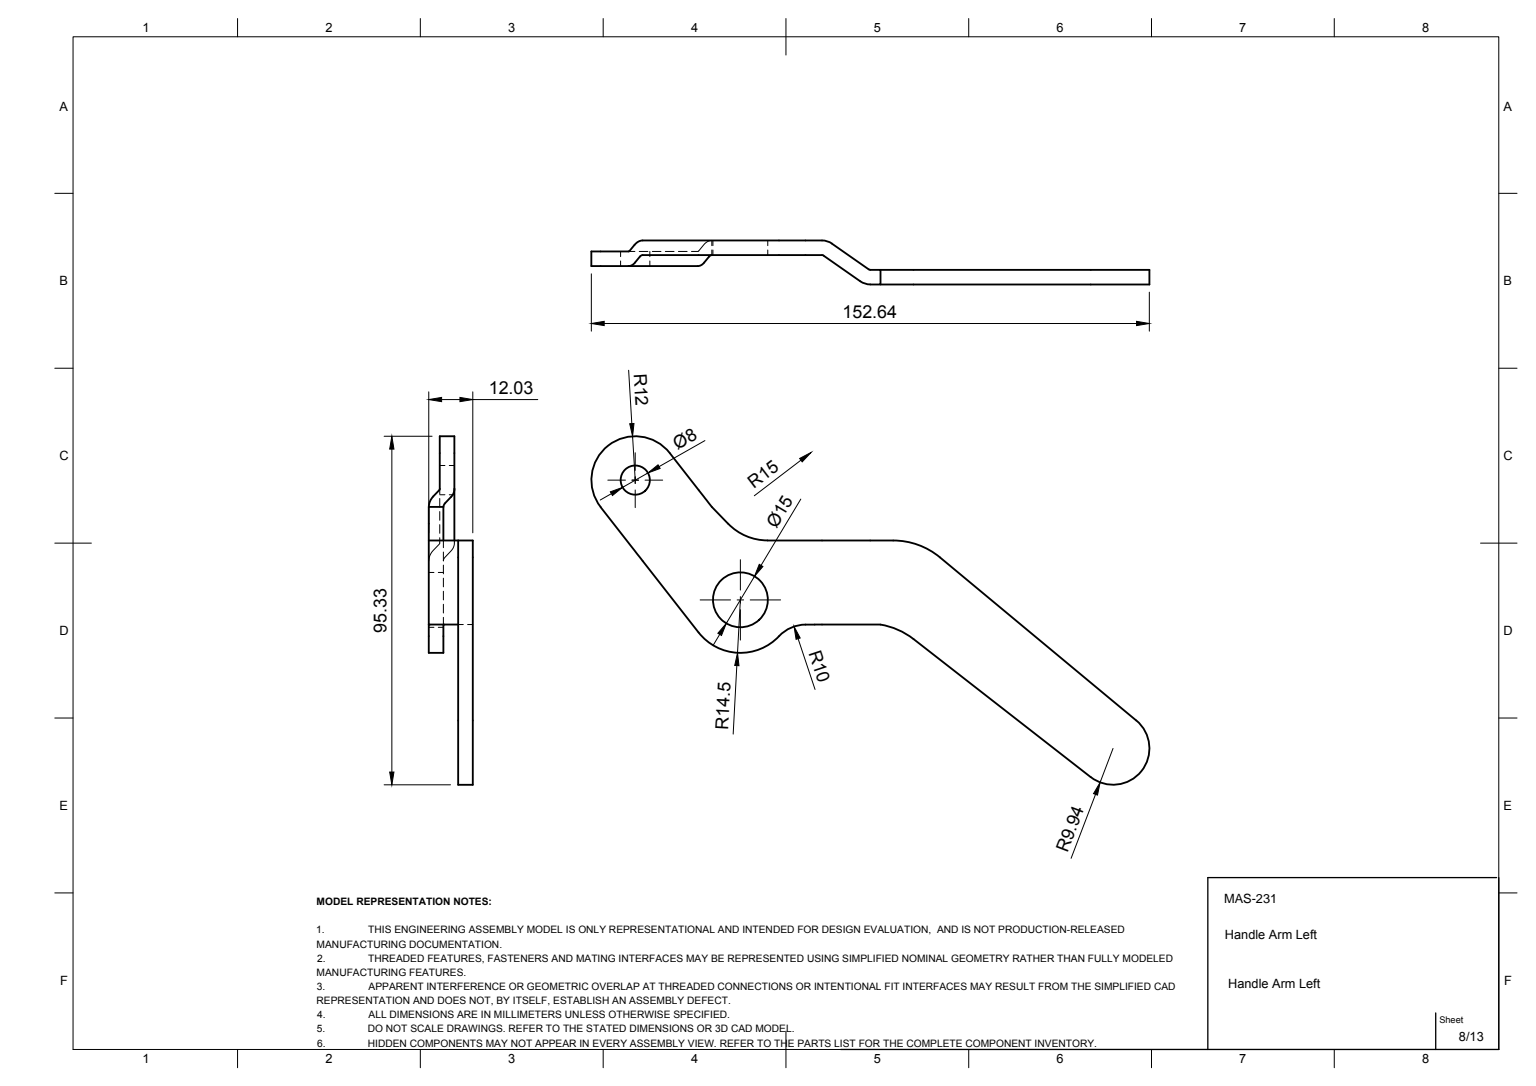
ISO-10303-21;
HEADER;
FILE_DESCRIPTION (('STEP AP214'),
    '1' );
FILE_NAME ( 'Handle Arm Left.step', '2026-10-04T02:08:54', ( '' ), ( '' ), 'STEP AP214', 'Unspecified', '' );
FILE_SCHEMA (( 'AUTOMOTIVE_DESIGN' ));
ENDSEC;
DATA;
#122=AXIS2_PLACEMENT_3D ( 'NONE', #43059, #39470, #7131 ) ;
#126=EDGE_LOOP ( 'NONE', ( #4193, #39037, #39203, #47364, #17831, #33692, #29299, #33986, #26594 ) ) ;
#187=( GEOMETRIC_REPRESENTATION_CONTEXT ( 3 ) GLOBAL_UNCERTAINTY_ASSIGNED_CONTEXT ( ( #19281 ) ) GLOBAL_UNIT_ASSIGNED_CONTEXT ( ( #14903, #26165, #18708 ) ) REPRESENTATION_CONTEXT ( 'NONE', 'WORKASPACE' ) ) ;
#223=EDGE_LOOP ( 'NONE', ( #32593, #34812, #29678, #45510 ) ) ;
#230=FACE_OUTER_BOUND ( 'NONE', #13816, .T. ) ;
#248=CARTESIAN_POINT ( 'NONE',  ( -0.3161444924769509779, 1.495705267341512767, -0.3569552279982057819 ) ) ;
#378=EDGE_CURVE ( 'NONE', #9213, #13081, #13737, .T. ) ;
#388=B_SPLINE_CURVE_WITH_KNOTS ( 'NONE', 3,
 ( #34639, #1791, #24318, #31755 ),
 .UNSPECIFIED., .F., .F.,
 ( 4, 4 ),
 ( 0.000000000000000000, 1.000000000000000000 ),
 .UNSPECIFIED. ) ;
#405=EDGE_CURVE ( 'NONE', #45750, #40086, #43961, .T. ) ;
#408=DIRECTION ( 'NONE',  ( -1.000000000000000000, 0.000000000000000000, 0.000000000000000000 ) ) ;
#422=VECTOR ( 'NONE', #8785, 39.37007874015748143 ) ;
#427=AXIS2_PLACEMENT_3D ( 'NONE', #21003, #3022, #14070 ) ;
#459=ORIENTED_EDGE ( 'NONE', *, *, #45696, .T. ) ;
#467=CARTESIAN_POINT ( 'NONE',  ( -0.07874015748031489015, -0.5708661417322835607, 0.9783464566929127582 ) ) ;
#518=CYLINDRICAL_SURFACE ( 'NONE', #9417, 0.5708661417322833387 ) ;
#533=EDGE_LOOP ( 'NONE', ( #23473, #14540, #33151, #19710 ) ) ;
#535=DIRECTION ( 'NONE',  ( 1.000000000000000000, -0.000000000000000000, -0.000000000000000000 ) ) ;
#539=CARTESIAN_POINT ( 'NONE',  ( -0.1586641775163213364, 1.209494567139720367, -1.479906699140297599 ) ) ;
#545=DIRECTION ( 'NONE',  ( 0.000000000000000000, -8.673617379884043361E-16, 1.000000000000000000 ) ) ;
#558=CARTESIAN_POINT ( 'NONE',  ( -0.1586641775163213364, 1.205832402325951680, -1.129708666049261900 ) ) ;
#616=ORIENTED_EDGE ( 'NONE', *, *, #20566, .T. ) ;
#679=FACE_OUTER_BOUND ( 'NONE', #47350, .T. ) ;
#696=AXIS2_PLACEMENT_3D ( 'NONE', #10327, #39534, #28800 ) ;
#711=AXIS2_PLACEMENT_3D ( 'NONE', #7841, #43130, #8307 ) ;
#753=EDGE_CURVE ( 'NONE', #41392, #4833, #15522, .T. ) ;
#754=PRODUCT_DEFINITION ( 'UNKNOWN', '', #15557, #11115 ) ;
#808=FACE_OUTER_BOUND ( 'NONE', #31107, .T. ) ;
#881=CARTESIAN_POINT ( 'NONE',  ( 0.1574803149606299746, 0.6241017553149654784, 0.3240160679609099259 ) ) ;
#895=CIRCLE ( 'NONE', #27749, 0.4724409448818896462 ) ;
#923=ORIENTED_EDGE ( 'NONE', *, *, #43493, .T. ) ;
#1025=ADVANCED_FACE ( 'NONE', ( #22928 ), #19568, .F. ) ;
#1029=LENGTH_MEASURE_WITH_UNIT ( LENGTH_MEASURE( 0.02539999999999999897 ), #18778 ) ;
#1037=CARTESIAN_POINT ( 'NONE',  ( -0.1184675242425147629, -0.09842519685039370636, 1.713085361781126803 ) ) ;
#1140=CARTESIAN_POINT ( 'NONE',  ( -0.3161444924769509779, 1.205832402325951680, -1.129708666049261900 ) ) ;
#1216=LINE ( 'NONE', #15633, #39726 ) ;
#1222=ORIENTED_EDGE ( 'NONE', *, *, #15124, .F. ) ;
#1296=DIRECTION ( 'NONE',  ( -0.000000000000000000, -0.2432573283306819767, 0.9699617890481142535 ) ) ;
#1309=VECTOR ( 'NONE', #45246, 39.37007874015748143 ) ;
#1316=DIRECTION ( 'NONE',  ( 0.000000000000000000, 0.000000000000000000, 1.000000000000000000 ) ) ;
#1330=LINE ( 'NONE', #2050, #12163 ) ;
#1374=DIRECTION ( 'NONE',  ( -1.000000000000000000, 0.000000000000000000, 0.000000000000000000 ) ) ;
#1393=DIRECTION ( 'NONE',  ( 0.000000000000000000, -1.000000000000000000, 0.000000000000000000 ) ) ;
#1444=EDGE_CURVE ( 'NONE', #18796, #17177, #32922, .T. ) ;
#1488=AXIS2_PLACEMENT_3D ( 'NONE', #8603, #23243, #19630 ) ;
#1493=VECTOR ( 'NONE', #28318, 39.37007874015748143 ) ;
#1494=EDGE_CURVE ( 'NONE', #3991, #16648, #40415, .T. ) ;
#1507=CARTESIAN_POINT ( 'NONE',  ( 0.03901279071809810040, -0.09842519685039370636, 1.870565676741754668 ) ) ;
#1532=EDGE_LOOP ( 'NONE', ( #26230, #3600, #16284, #44821 ) ) ;
#1601=AXIS2_PLACEMENT_3D ( 'NONE', #34251, #4042, #22736 ) ;
#1613=DIRECTION ( 'NONE',  ( 1.000000000000000000, -0.000000000000000000, -0.000000000000000000 ) ) ;
#1634=DIRECTION ( 'NONE',  ( 0.000000000000000000, 0.000000000000000000, 1.000000000000000000 ) ) ;
#1791=CARTESIAN_POINT ( 'NONE',  ( 0.1049868766404236653, 0.4668427075568369333, -0.7022306805398673690 ) ) ;
#1868=DIRECTION ( 'NONE',  ( -0.8191520442890007914, -0.4519843998600331925, 0.3531289150159138690 ) ) ;
#1878=DIRECTION ( 'NONE',  ( 0.000000000000000000, -1.000000000000000000, 0.000000000000000000 ) ) ;
#1947=EDGE_CURVE ( 'NONE', #45939, #23245, #19092, .T. ) ;
#1972=AXIS2_PLACEMENT_3D ( 'NONE', #43308, #35675, #44016 ) ;
#1994=EDGE_CURVE ( 'NONE', #30756, #31965, #2268, .T. ) ;
#2006=ORIENTED_EDGE ( 'NONE', *, *, #33798, .F. ) ;
#2044=DIRECTION ( 'NONE',  ( 0.000000000000000000, 0.000000000000000000, -1.000000000000000000 ) ) ;
#2050=CARTESIAN_POINT ( 'NONE',  ( -0.3161444924769509779, 0.8918838478058892516, -1.034309214090478823 ) ) ;
#2090=ORIENTED_EDGE ( 'NONE', *, *, #33751, .T. ) ;
#2145=DIRECTION ( 'NONE',  ( 0.000000000000000000, 0.000000000000000000, 1.000000000000000000 ) ) ;
#2163=LINE ( 'NONE', #46478, #34704 ) ;
#2207=LINE ( 'NONE', #37047, #4035 ) ;
#2248=ORIENTED_EDGE ( 'NONE', *, *, #47327, .F. ) ;
#2268=CIRCLE ( 'NONE', #24483, 0.2952755905511806334 ) ;
#2320=EDGE_CURVE ( 'NONE', #11282, #39413, #6695, .T. ) ;
#2339=CARTESIAN_POINT ( 'NONE',  ( -0.1586641775163213364, 1.975221432870719385, -0.9622519263226601005 ) ) ;
#2340=DIRECTION ( 'NONE',  ( 1.000000000000000000, -0.000000000000000000, -0.000000000000000000 ) ) ;
#2345=CARTESIAN_POINT ( 'NONE',  ( -0.3161444924769509779, 0.1169123912647635627, -2.121729632260043186 ) ) ;
#2392=DIRECTION ( 'NONE',  ( 1.000000000000000000, 0.000000000000000000, 0.000000000000000000 ) ) ;
#2463=CARTESIAN_POINT ( 'NONE',  ( 0.000000000000000000, 0.3740157480314960647, 0.9783464566929134243 ) ) ;
#2465=ORIENTED_EDGE ( 'NONE', *, *, #15820, .T. ) ;
#2494=ORIENTED_EDGE ( 'NONE', *, *, #12903, .T. ) ;
#2497=CARTESIAN_POINT ( 'NONE',  ( -0.3161444924769509779, 1.025704337919491005, -1.138861239548321524 ) ) ;
#2575=DIRECTION ( 'NONE',  ( 0.000000000000000000, 0.000000000000000000, -1.000000000000000000 ) ) ;
#2644=EDGE_CURVE ( 'NONE', #46787, #41828, #31616, .T. ) ;
#2652=ORIENTED_EDGE ( 'NONE', *, *, #33847, .T. ) ;
#2664=CARTESIAN_POINT ( 'NONE',  ( 0.1574803149606299746, 3.616083068348478250E-17, 0.2952755905511806334 ) ) ;
#2710=EDGE_CURVE ( 'NONE', #3855, #15659, #13395, .T. ) ;
#2751=ORIENTED_EDGE ( 'NONE', *, *, #19643, .T. ) ;
#2914=PLANE ( 'NONE',  #36780 ) ;
#3012=VERTEX_POINT ( 'NONE', #33217 ) ;
#3022=DIRECTION ( 'NONE',  ( 0.8191520442890009024, 0.4519843998600359125, -0.3531289150159101498 ) ) ;
#3029=LINE ( 'NONE', #24857, #4888 ) ;
#3049=CARTESIAN_POINT ( 'NONE',  ( 0.1574803149606339714, 0.5288907983920063671, -0.7507079620615686455 ) ) ;
#3060=VERTEX_POINT ( 'NONE', #33447 ) ;
#3071=DIRECTION ( 'NONE',  ( -1.000000000000000000, 0.000000000000000000, 0.000000000000000000 ) ) ;
#3105=VERTEX_POINT ( 'NONE', #14329 ) ;
#3185=DIRECTION ( 'NONE',  ( -1.000000000000000000, 0.000000000000000000, 0.000000000000000000 ) ) ;
#3230=ORIENTED_EDGE ( 'NONE', *, *, #31890, .T. ) ;
#3258=AXIS2_PLACEMENT_3D ( 'NONE', #29797, #27075, #45706 ) ;
#3268=EDGE_CURVE ( 'NONE', #3438, #30045, #43775, .T. ) ;
#3269=FACE_OUTER_BOUND ( 'NONE', #7093, .T. ) ;
#3302=CARTESIAN_POINT ( 'NONE',  ( -0.07874015748031495954, 0.3740157480314960092, 0.9783464566929293005 ) ) ;
#3367=ORIENTED_EDGE ( 'NONE', *, *, #44807, .F. ) ;
#3377=LINE ( 'NONE', #36680, #16947 ) ;
#3382=CARTESIAN_POINT ( 'NONE',  ( -0.1586641775163213364, 1.975221432870719385, -0.9622519263226598785 ) ) ;
#3389=ORIENTED_EDGE ( 'NONE', *, *, #24381, .T. ) ;
#3438=VERTEX_POINT ( 'NONE', #8769 ) ;
#3503=ORIENTED_EDGE ( 'NONE', *, *, #37106, .T. ) ;
#3510=ORIENTED_EDGE ( 'NONE', *, *, #33798, .T. ) ;
#3600=ORIENTED_EDGE ( 'NONE', *, *, #47358, .T. ) ;
#3602=ORIENTED_EDGE ( 'NONE', *, *, #47057, .T. ) ;
#3676=DIRECTION ( 'NONE',  ( -1.000000000000000000, 0.000000000000000000, 0.000000000000000000 ) ) ;
#3692=EDGE_CURVE ( 'NONE', #30045, #26635, #32407, .T. ) ;
#3726=CARTESIAN_POINT ( 'NONE',  ( 0.000000000000000000, 0.000000000000000000, 0.000000000000000000 ) ) ;
#3810=CARTESIAN_POINT ( 'NONE',  ( -0.1586641775163213364, 2.559880088878760951, -3.648497683167374550 ) ) ;
#3839=VECTOR ( 'NONE', #5194, 39.37007874015748143 ) ;
#3855=VERTEX_POINT ( 'NONE', #13599 ) ;
#3877=FACE_OUTER_BOUND ( 'NONE', #1532, .T. ) ;
#3896=ADVANCED_FACE ( 'NONE', ( #24175 ), #42358, .F. ) ;
#3911=ORIENTED_EDGE ( 'NONE', *, *, #13388, .T. ) ;
#3950=ADVANCED_FACE ( 'NONE', ( #21260 ), #39689, .F. ) ;
#3984=VECTOR ( 'NONE', #43167, 39.37007874015748143 ) ;
#3991=VERTEX_POINT ( 'NONE', #22424 ) ;
#3992=EDGE_CURVE ( 'NONE', #35281, #23980, #2207, .T. ) ;
#4012=CARTESIAN_POINT ( 'NONE',  ( -0.02899999999999994943, 0.5288907983920058120, -0.7507079620615694227 ) ) ;
#4035=VECTOR ( 'NONE', #37518, 39.37007874015748854 ) ;
#4040=ORIENTED_EDGE ( 'NONE', *, *, #27793, .F. ) ;
#4042=DIRECTION ( 'NONE',  ( -1.000000000000000000, 0.000000000000000000, 0.000000000000000000 ) ) ;
#4044=CARTESIAN_POINT ( 'NONE',  ( 0.1574803149606299746, 0.1473293504822046074, -0.5595480905233950475 ) ) ;
#4081=FACE_OUTER_BOUND ( 'NONE', #15189, .T. ) ;
#4125=LINE ( 'NONE', #8196, #30626 ) ;
#4152=PRESENTATION_STYLE_ASSIGNMENT (( #37229 ) ) ;
#4193=ORIENTED_EDGE ( 'NONE', *, *, #17844, .F. ) ;
#4301=ORIENTED_EDGE ( 'NONE', *, *, #47118, .T. ) ;
#4305=ORIENTED_EDGE ( 'NONE', *, *, #13909, .F. ) ;
#4425=ADVANCED_FACE ( 'NONE', ( #36701 ), #15141, .T. ) ;
#4491=VERTEX_POINT ( 'NONE', #44335 ) ;
#4518=ORIENTED_EDGE ( 'NONE', *, *, #44084, .T. ) ;
#4566=VECTOR ( 'NONE', #29486, 39.37007874015748143 ) ;
#4593=VECTOR ( 'NONE', #29577, 39.37007874015748143 ) ;
#4665=CARTESIAN_POINT ( 'NONE',  ( 0.06801279071809869514, -0.09842519685039370636, 1.224299699984025658 ) ) ;
#4719=DIRECTION ( 'NONE',  ( -0.5735764363510332808, 0.6455006197386625733, -0.5043203561029951931 ) ) ;
#4750=EDGE_CURVE ( 'NONE', #18385, #41392, #9600, .T. ) ;
#4784=DIRECTION ( 'NONE',  ( 0.000000000000000000, -1.000000000000000000, 0.000000000000000000 ) ) ;
#4797=DIRECTION ( 'NONE',  ( -1.000000000000000000, 0.000000000000000000, 0.000000000000000000 ) ) ;
#4801=EDGE_CURVE ( 'NONE', #39413, #16648, #39040, .T. ) ;
#4802=VECTOR ( 'NONE', #26824, 39.37007874015748143 ) ;
#4833=VERTEX_POINT ( 'NONE', #20600 ) ;
#4888=VECTOR ( 'NONE', #35420, 39.37007874015748143 ) ;
#4916=CARTESIAN_POINT ( 'NONE',  ( 0.000000000000000000, -0.5708661417322835607, -6.991093932140394160E-17 ) ) ;
#4920=CIRCLE ( 'NONE', #41633, 0.3937007874015748254 ) ;
#4952=AXIS2_PLACEMENT_3D ( 'NONE', #19826, #34454, #34939 ) ;
#4984=VECTOR ( 'NONE', #6909, 39.37007874015748143 ) ;
#4990=CIRCLE ( 'NONE', #21061, 0.5905511811023623769 ) ;
#5011=DIRECTION ( 'NONE',  ( 0.000000000000000000, -0.7880107536067216811, 0.6156614753256587358 ) ) ;
#5016=ORIENTED_EDGE ( 'NONE', *, *, #12269, .T. ) ;
#5131=ORIENTED_EDGE ( 'NONE', *, *, #12269, .F. ) ;
#5151=ORIENTED_EDGE ( 'NONE', *, *, #40888, .F. ) ;
#5160=DIRECTION ( 'NONE',  ( -0.000000000000000000, -0.000000000000000000, -1.000000000000000000 ) ) ;
#5161=CARTESIAN_POINT ( 'NONE',  ( -0.1586641775163213364, 0.4457451269443606368, -1.671447902550282194 ) ) ;
#5189=ADVANCED_FACE ( 'NONE', ( #21246 ), #28719, .T. ) ;
#5194=DIRECTION ( 'NONE',  ( -1.000000000000000000, 0.000000000000000000, 0.000000000000000000 ) ) ;
#5242=VECTOR ( 'NONE', #12954, 39.37007874015748143 ) ;
#5252=EDGE_LOOP ( 'NONE', ( #21164, #13883, #3389, #45534 ) ) ;
#5272=ORIENTED_EDGE ( 'NONE', *, *, #15550, .T. ) ;
#5276=CIRCLE ( 'NONE', #29028, 0.1574803149606292529 ) ;
#5330=VECTOR ( 'NONE', #16587, 39.37007874015748854 ) ;
#5442=DIRECTION ( 'NONE',  ( 0.000000000000000000, -0.7880107536067203489, 0.6156614753256604011 ) ) ;
#5457=ORIENTED_EDGE ( 'NONE', *, *, #1947, .F. ) ;
#5464=DIRECTION ( 'NONE',  ( 1.000000000000000000, -0.000000000000000000, -0.000000000000000000 ) ) ;
#5467=CARTESIAN_POINT ( 'NONE',  ( -0.3161444924769509779, 1.975221432870719385, -0.9622519263226598785 ) ) ;
#5499=DIRECTION ( 'NONE',  ( 0.000000000000000000, 0.6156614753256605121, 0.7880107536067204599 ) ) ;
#5512=ORIENTED_EDGE ( 'NONE', *, *, #18930, .F. ) ;
#5556=ORIENTED_EDGE ( 'NONE', *, *, #9114, .T. ) ;
#5658=AXIS2_PLACEMENT_3D ( 'NONE', #22546, #40967, #25919 ) ;
#5685=VERTEX_POINT ( 'NONE', #3382 ) ;
#5710=DIRECTION ( 'NONE',  ( 0.5735764363510332808, -0.6455006197386625733, 0.5043203561029951931 ) ) ;
#5752=AXIS2_PLACEMENT_3D ( 'NONE', #39780, #21596, #36232 ) ;
#5792=CARTESIAN_POINT ( 'NONE',  ( 0.1574803149606299746, 0.3740157480314960647, 1.057384721142220263 ) ) ;
#5806=LINE ( 'NONE', #35751, #39943 ) ;
#5917=VERTEX_POINT ( 'NONE', #881 ) ;
#5935=DIRECTION ( 'NONE',  ( 0.000000000000000000, -0.7880107536067214591, 0.6156614753256588468 ) ) ;
#5954=ORIENTED_EDGE ( 'NONE', *, *, #753, .F. ) ;
#5960=CARTESIAN_POINT ( 'NONE',  ( -0.1296641775163210608, 1.495705267341510769, -0.3569552279982081133 ) ) ;
#5968=DIRECTION ( 'NONE',  ( 0.000000000000000000, 0.000000000000000000, -1.000000000000000000 ) ) ;
#5972=CARTESIAN_POINT ( 'NONE',  ( 0.1574803149606299746, 0.1473293504822046074, -0.9532488779249699284 ) ) ;
#5988=AXIS2_PLACEMENT_3D ( 'NONE', #23729, #4784, #19885 ) ;
#6038=VECTOR ( 'NONE', #12574, 39.37007874015748143 ) ;
#6078=CARTESIAN_POINT ( 'NONE',  ( 0.1574803149606299746, 0.6926248950869623444, -0.5411378750921671532 ) ) ;
#6123=EDGE_LOOP ( 'NONE', ( #40691, #27689, #20849, #42886 ) ) ;
#6147=EDGE_CURVE ( 'NONE', #36995, #3438, #34129, .T. ) ;
#6149=CARTESIAN_POINT ( 'NONE',  ( 0.1574803149606300023, 0.000000000000000000, 0.000000000000000000 ) ) ;
#6166=CARTESIAN_POINT ( 'NONE',  ( -0.2824199087359777760, 1.411419074098319903, -0.2911036367043356443 ) ) ;
#6200=DIRECTION ( 'NONE',  ( -1.000000000000000000, -0.000000000000000000, -0.000000000000000000 ) ) ;
#6201=ORIENTED_EDGE ( 'NONE', *, *, #1444, .F. ) ;
#6206=DIRECTION ( 'NONE',  ( -0.000000000000000000, -0.000000000000000000, 1.000000000000000000 ) ) ;
#6263=ADVANCED_FACE ( 'NONE', ( #22896 ), #21955, .F. ) ;
#6378=VERTEX_POINT ( 'NONE', #37753 ) ;
#6391=DIRECTION ( 'NONE',  ( 0.000000000000000000, 0.000000000000000000, -1.000000000000000000 ) ) ;
#6400=CARTESIAN_POINT ( 'NONE',  ( 0.1099139000111727937, 0.3740157480314960647, 1.120507485783946100 ) ) ;
#6436=VECTOR ( 'NONE', #6206, 39.37007874015748143 ) ;
#6595=EDGE_LOOP ( 'NONE', ( #9256, #30277, #9094, #9082 ) ) ;
#6671=CARTESIAN_POINT ( 'NONE',  ( 0.1574803149606299746, 0.3740157480314960647, 0.9783464566929134243 ) ) ;
#6695=LINE ( 'NONE', #21311, #32152 ) ;
#6697=VECTOR ( 'NONE', #42238, 39.37007874015748143 ) ;
#6734=LINE ( 'NONE', #2664, #33870 ) ;
#6735=ORIENTED_EDGE ( 'NONE', *, *, #15124, .T. ) ;
#6823=ORIENTED_EDGE ( 'NONE', *, *, #40550, .T. ) ;
#6824=DIRECTION ( 'NONE',  ( 0.000000000000000000, 0.6156614753256605121, 0.7880107536067204599 ) ) ;
#6847=DIRECTION ( 'NONE',  ( -0.000000000000000000, -0.6156614753256605121, -0.7880107536067204599 ) ) ;
#6861=CARTESIAN_POINT ( 'NONE',  ( -0.07874015748031495954, -0.5708661417322833387, 0.9783464566929284123 ) ) ;
#6876=DIRECTION ( 'NONE',  ( 0.000000000000000000, -0.7880107536067239016, 0.6156614753256557382 ) ) ;
#6877=LINE ( 'NONE', #2339, #41152 ) ;
#6909=DIRECTION ( 'NONE',  ( 0.000000000000000000, -0.6156614753256639538, -0.7880107536067174623 ) ) ;
#6911=AXIS2_PLACEMENT_3D ( 'NONE', #23945, #1878, #2575 ) ;
#6924=CARTESIAN_POINT ( 'NONE',  ( 1.530041696156790562E-15, 0.4667239666988196034, -0.7023826619074857724 ) ) ;
#7001=DIRECTION ( 'NONE',  ( 1.000000000000000000, -0.000000000000000000, -0.000000000000000000 ) ) ;
#7009=AXIS2_PLACEMENT_3D ( 'NONE', #23522, #11797, #19432 ) ;
#7087=ORIENTED_EDGE ( 'NONE', *, *, #2710, .T. ) ;
#7093=EDGE_LOOP ( 'NONE', ( #26363, #18372, #16064, #13224 ) ) ;
#7131=DIRECTION ( 'NONE',  ( 0.000000000000000000, 3.556183125752454544E-15, 1.000000000000000000 ) ) ;
#7162=VERTEX_POINT ( 'NONE', #2497 ) ;
#7410=DIRECTION ( 'NONE',  ( -1.000000000000000000, 0.000000000000000000, 0.000000000000000000 ) ) ;
#7415=VERTEX_POINT ( 'NONE', #18067 ) ;
#7480=PLANE ( 'NONE',  #36037 ) ;
#7567=ORIENTED_EDGE ( 'NONE', *, *, #14071, .F. ) ;
#7706=CARTESIAN_POINT ( 'NONE',  ( 0.1574803149606299746, 0.000000000000000000, 0.000000000000000000 ) ) ;
#7768=ADVANCED_FACE ( 'NONE', ( #41413, #230 ), #7904, .T. ) ;
#7828=ADVANCED_BREP_SHAPE_REPRESENTATION ( 'Handle Arm Left', ( #36032, #20860 ), #187 ) ;
#7841=CARTESIAN_POINT ( 'NONE',  ( 0.1574803149606299746, -5.122214988120488358E-16, -8.878505979408856939E-16 ) ) ;
#7874=DIRECTION ( 'NONE',  ( 1.000000000000000000, -0.000000000000000000, -0.000000000000000000 ) ) ;
#7904=PLANE ( 'NONE',  #40908 ) ;
#8038=ORIENTED_EDGE ( 'NONE', *, *, #14363, .T. ) ;
#8046=LINE ( 'NONE', #23151, #41459 ) ;
#8071=CARTESIAN_POINT ( 'NONE',  ( 0.04485236092672649499, -0.5708661417322835607, 1.206847064312615903 ) ) ;
#8084=CYLINDRICAL_SURFACE ( 'NONE', #24731, 0.1864803149606299171 ) ;
#8096=EDGE_LOOP ( 'NONE', ( #32413, #41131 ) ) ;
#8110=LINE ( 'NONE', #24976, #39050 ) ;
#8196=CARTESIAN_POINT ( 'NONE',  ( 0.000000000000000000, 0.3740157480314960647, 0.9783464566929134243 ) ) ;
#8235=DIRECTION ( 'NONE',  ( 0.000000000000000000, -0.7880107536067215701, 0.6156614753256588468 ) ) ;
#8307=DIRECTION ( 'NONE',  ( 0.000000000000000000, 0.000000000000000000, 1.000000000000000000 ) ) ;
#8336=EDGE_CURVE ( 'NONE', #39972, #13132, #18470, .T. ) ;
#8343=AXIS2_PLACEMENT_3D ( 'NONE', #13965, #43413, #10622 ) ;
#8347=LINE ( 'NONE', #15570, #4802 ) ;
#8370=ORIENTED_EDGE ( 'NONE', *, *, #4801, .F. ) ;
#8438=ORIENTED_EDGE ( 'NONE', *, *, #18015, .T. ) ;
#8441=FACE_OUTER_BOUND ( 'NONE', #9696, .T. ) ;
#8489=ADVANCED_FACE ( 'NONE', ( #4081 ), #28823, .F. ) ;
#8539=CARTESIAN_POINT ( 'NONE',  ( -0.02900000000000056352, 1.086379535891625059, -0.03715491745705514631 ) ) ;
#8563=LINE ( 'NONE', #38275, #24910 ) ;
#8603=CARTESIAN_POINT ( 'NONE',  ( -0.02899999999999994943, 0.5288907983920065892, -0.7507079620615685345 ) ) ;
#8613=DIRECTION ( 'NONE',  ( 0.000000000000000000, -1.000000000000000000, 0.000000000000000000 ) ) ;
#8696=ADVANCED_FACE ( 'NONE', ( #26868 ), #31412, .F. ) ;
#8749=VERTEX_POINT ( 'NONE', #30945 ) ;
#8769=CARTESIAN_POINT ( 'NONE',  ( -0.1586641775163213364, 1.495705267341508771, -0.3569552279982025622 ) ) ;
#8785=DIRECTION ( 'NONE',  ( 1.000000000000000000, -0.000000000000000000, -0.000000000000000000 ) ) ;
#8956=DIRECTION ( 'NONE',  ( 0.000000000000000000, 0.7880107536067179064, -0.6156614753256635098 ) ) ;
#9018=DIRECTION ( 'NONE',  ( 0.000000000000000000, -0.6156614753256639538, -0.7880107536067174623 ) ) ;
#9046=FACE_OUTER_BOUND ( 'NONE', #25909, .T. ) ;
#9066=LINE ( 'NONE', #45698, #16335 ) ;
#9082=ORIENTED_EDGE ( 'NONE', *, *, #3992, .T. ) ;
#9088=AXIS2_PLACEMENT_3D ( 'NONE', #17462, #3071, #5968 ) ;
#9094=ORIENTED_EDGE ( 'NONE', *, *, #23438, .T. ) ;
#9114=EDGE_CURVE ( 'NONE', #13081, #26397, #17703, .T. ) ;
#9151=CARTESIAN_POINT ( 'NONE',  ( -0.1184675242425147629, -0.5708661417322835607, 1.161904259418922170 ) ) ;
#9198=ORIENTED_EDGE ( 'NONE', *, *, #12903, .F. ) ;
#9213=VERTEX_POINT ( 'NONE', #15072 ) ;
#9256=ORIENTED_EDGE ( 'NONE', *, *, #44505, .F. ) ;
#9308=CARTESIAN_POINT ( 'NONE',  ( -0.3161444924769509779, 1.449372585305507943, -0.3207561694859686896 ) ) ;
#9324=CYLINDRICAL_SURFACE ( 'NONE', #6911, 0.2362204724409448231 ) ;
#9417=AXIS2_PLACEMENT_3D ( 'NONE', #29370, #3185, #14231 ) ;
#9422=VECTOR ( 'NONE', #20147, 39.37007874015748854 ) ;
#9441=CARTESIAN_POINT ( 'NONE',  ( 3.060083392313581123E-15, 0.9310112235910578127, -1.064878870394357468 ) ) ;
#9491=EDGE_CURVE ( 'NONE', #9213, #5917, #45332, .T. ) ;
#9526=EDGE_LOOP ( 'NONE', ( #34107, #20828 ) ) ;
#9600=LINE ( 'NONE', #9833, #24085 ) ;
#9647=CARTESIAN_POINT ( 'NONE',  ( 0.1574803149606319730, 0.4667239666988196034, -0.7023826619074858835 ) ) ;
#9696=EDGE_LOOP ( 'NONE', ( #2494, #36190, #1222, #13297 ) ) ;
#9701=VERTEX_POINT ( 'NONE', #36101 ) ;
#9705=LINE ( 'NONE', #6078, #36691 ) ;
#9707=ORIENTED_EDGE ( 'NONE', *, *, #36916, .F. ) ;
#9725=DIRECTION ( 'NONE',  ( 0.000000000000000000, 0.7907053606985338101, -0.6121968903568536513 ) ) ;
#9819=ADVANCED_FACE ( 'NONE', ( #8441 ), #41236, .T. ) ;
#9833=CARTESIAN_POINT ( 'NONE',  ( -0.3161444924769509779, 2.559880088878760951, -3.648497683167374550 ) ) ;
#9894=LINE ( 'NONE', #25470, #28521 ) ;
#9936=CIRCLE ( 'NONE', #36707, 0.02900000000000062597 ) ;
#10106=AXIS2_PLACEMENT_3D ( 'NONE', #25599, #17436, #17672 ) ;
#10117=CARTESIAN_POINT ( 'NONE',  ( 0.000000000000000000, 0.9876813667277571929, 0.7893767492247212303 ) ) ;
#10122=EDGE_CURVE ( 'NONE', #9701, #18496, #26607, .T. ) ;
#10199=MECHANICAL_DESIGN_GEOMETRIC_PRESENTATION_REPRESENTATION('',(#25515),#31637);
#10265=DIRECTION ( 'NONE',  ( 1.000000000000000000, 0.000000000000000000, -0.000000000000000000 ) ) ;
#10268=VERTEX_POINT ( 'NONE', #3049 ) ;
#10278=ORIENTED_EDGE ( 'NONE', *, *, #6147, .T. ) ;
#10327=CARTESIAN_POINT ( 'NONE',  ( 0.1574803149606299746, 0.1473293504822046074, -0.9532488779249699284 ) ) ;
#10377=FACE_OUTER_BOUND ( 'NONE', #26749, .T. ) ;
#10398=DIRECTION ( 'NONE',  ( -1.000000000000000000, -0.000000000000000000, -0.000000000000000000 ) ) ;
#10444=CARTESIAN_POINT ( 'NONE',  ( 0.06801279071809869514, 0.3740157480314960647, 1.224299699984025658 ) ) ;
#10448=CARTESIAN_POINT ( 'NONE',  ( -0.02899999999999994943, 1.086379535891617509, -0.03715491745705647858 ) ) ;
#10454=CARTESIAN_POINT ( 'NONE',  ( -0.08091701073424917290, 0.3740157480314960647, 1.112073044918590048 ) ) ;
#10487=CYLINDRICAL_SURFACE ( 'NONE', #25712, 0.07874015748031489015 ) ;
#10497=VERTEX_POINT ( 'NONE', #22650 ) ;
#10501=DIRECTION ( 'NONE',  ( 1.217491584052838080E-15, 0.6156614753256588468, 0.7880107536067214591 ) ) ;
#10512=EDGE_CURVE ( 'NONE', #40086, #45750, #44935, .T. ) ;
#10522=ORIENTED_EDGE ( 'NONE', *, *, #44505, .T. ) ;
#10548=DIRECTION ( 'NONE',  ( 0.000000000000000000, 0.000000000000000000, 1.000000000000000000 ) ) ;
#10560=DIRECTION ( 'NONE',  ( 0.000000000000000000, 0.2126700594527842492, -0.9771240687918547607 ) ) ;
#10573=CARTESIAN_POINT ( 'NONE',  ( -0.1586641775163213364, 1.914733266569311532, -0.6843357808987579061 ) ) ;
#10580=EDGE_CURVE ( 'NONE', #3855, #8749, #44902, .T. ) ;
#10602=ORIENTED_EDGE ( 'NONE', *, *, #33847, .F. ) ;
#10622=DIRECTION ( 'NONE',  ( 0.000000000000000000, 0.000000000000000000, 1.000000000000000000 ) ) ;
#10651=CARTESIAN_POINT ( 'NONE',  ( 0.1574803149606299746, 0.9876813667277571929, 0.7893767492247212303 ) ) ;
#10669=DIRECTION ( 'NONE',  ( -0.000000000000000000, 0.000000000000000000, -1.000000000000000000 ) ) ;
#10715=CARTESIAN_POINT ( 'NONE',  ( -0.1296641775163207277, 1.495705267341506772, -0.3569552279982053378 ) ) ;
#10777=CARTESIAN_POINT ( 'NONE',  ( 0.000000000000000000, 0.6926248950869576815, -0.5411378750921725933 ) ) ;
#10801=AXIS2_PLACEMENT_3D ( 'NONE', #37533, #37781, #30158 ) ;
#10803=LINE ( 'NONE', #29032, #21582 ) ;
#10835=DIRECTION ( 'NONE',  ( 1.000000000000000000, 0.000000000000000000, 0.000000000000000000 ) ) ;
#10872=ORIENTED_EDGE ( 'NONE', *, *, #40538, .F. ) ;
#10957=ORIENTED_EDGE ( 'NONE', *, *, #3992, .F. ) ;
#10978=CARTESIAN_POINT ( 'NONE',  ( -0.1586641775163213364, 0.1169123912647608288, -2.121729632260068055 ) ) ;
#11030=CARTESIAN_POINT ( 'NONE',  ( -0.3161444924769509779, 2.559880088878760951, -3.648497683167374550 ) ) ;
#11033=CIRCLE ( 'NONE', #34035, 0.4724409448818896462 ) ;
#11115=PRODUCT_DEFINITION_CONTEXT ( 'detailed design', #26947, 'design' ) ;
#11137=AXIS2_PLACEMENT_3D ( 'NONE', #4665, #11189, #18583 ) ;
#11172=ORIENTED_EDGE ( 'NONE', *, *, #44084, .F. ) ;
#11186=ADVANCED_FACE ( 'NONE', ( #26498 ), #45135, .T. ) ;
#11189=DIRECTION ( 'NONE',  ( 0.000000000000000000, -1.000000000000000000, -0.000000000000000000 ) ) ;
#11206=CARTESIAN_POINT ( 'NONE',  ( 0.1574803149606299746, 0.08719492171395763769, -0.5641677032617172793 ) ) ;
#11209=DIRECTION ( 'NONE',  ( -0.000000000000000000, -0.6156614753256575145, -0.7880107536067225693 ) ) ;
#11267=ADVANCED_FACE ( 'NONE', ( #37252, #808 ), #16642, .T. ) ;
#11282=VERTEX_POINT ( 'NONE', #20925 ) ;
#11296=DIRECTION ( 'NONE',  ( 2.775557561562890735E-17, -0.6156614753256639538, -0.7880107536067174623 ) ) ;
#11335=FACE_OUTER_BOUND ( 'NONE', #21755, .T. ) ;
#11370=AXIS2_PLACEMENT_3D ( 'NONE', #39169, #38722, #17607 ) ;
#11407=ORIENTED_EDGE ( 'NONE', *, *, #15210, .F. ) ;
#11468=ORIENTED_EDGE ( 'NONE', *, *, #15210, .T. ) ;
#11500=DIRECTION ( 'NONE',  ( 0.000000000000000000, 0.000000000000000000, -1.000000000000000000 ) ) ;
#11501=DIRECTION ( 'NONE',  ( 0.000000000000000000, 0.9945218953682737340, 0.1045284632676499459 ) ) ;
#11611=( NAMED_UNIT ( * ) PLANE_ANGLE_UNIT ( ) SI_UNIT ( $, .RADIAN. ) ) ;
#11665=AXIS2_PLACEMENT_3D ( 'NONE', #10444, #32497, #29162 ) ;
#11759=VECTOR ( 'NONE', #4719, 39.37007874015747433 ) ;
#11783=ORIENTED_EDGE ( 'NONE', *, *, #1494, .T. ) ;
#11786=ORIENTED_EDGE ( 'NONE', *, *, #44329, .F. ) ;
#11797=DIRECTION ( 'NONE',  ( -0.000000000000000000, 1.000000000000000000, -0.000000000000000000 ) ) ;
#11830=ORIENTED_EDGE ( 'NONE', *, *, #9491, .F. ) ;
#11848=AXIS2_PLACEMENT_3D ( 'NONE', #5161, #22430, #24556 ) ;
#11885=EDGE_CURVE ( 'NONE', #4491, #9701, #47296, .T. ) ;
#11976=LINE ( 'NONE', #4044, #25875 ) ;
#11983=CYLINDRICAL_SURFACE ( 'NONE', #26456, 0.5905511811023623769 ) ;
#11990=UNCERTAINTY_MEASURE_WITH_UNIT (LENGTH_MEASURE( 1.000000000000000082E-05 ), #45107, 'distance_accuracy_value', 'NONE') ;
#12022=CARTESIAN_POINT ( 'NONE',  ( -0.1184675242425147629, -0.5708661417322835607, 1.224299699984019885 ) ) ;
#12037=CARTESIAN_POINT ( 'NONE',  ( -0.1586641775163213364, 0.8918838478058892516, -1.034309214090478823 ) ) ;
#12059=ORIENTED_EDGE ( 'NONE', *, *, #23070, .T. ) ;
#12071=VECTOR ( 'NONE', #1296, 39.37007874015748854 ) ;
#12131=ORIENTED_EDGE ( 'NONE', *, *, #26787, .T. ) ;
#12163=VECTOR ( 'NONE', #23406, 39.37007874015748854 ) ;
#12173=LINE ( 'NONE', #26797, #11759 ) ;
#12269=EDGE_CURVE ( 'NONE', #41828, #39972, #22070, .T. ) ;
#12352=DIRECTION ( 'NONE',  ( 0.000000000000000000, 0.000000000000000000, 1.000000000000000000 ) ) ;
#12363=VECTOR ( 'NONE', #16978, 39.37007874015748143 ) ;
#12439=CYLINDRICAL_SURFACE ( 'NONE', #29320, 0.7874015748031496509 ) ;
#12452=DIRECTION ( 'NONE',  ( -0.5735764363510331698, 0.6455006197386586875, -0.5043203561029997450 ) ) ;
#12459=CARTESIAN_POINT ( 'NONE',  ( -0.3161444924769509779, 1.690605217543008632, -0.5092277576975117181 ) ) ;
#12465=ORIENTED_EDGE ( 'NONE', *, *, #31141, .T. ) ;
#12495=ADVANCED_FACE ( 'NONE', ( #43863 ), #27116, .T. ) ;
#12519=CARTESIAN_POINT ( 'NONE',  ( 0.5785143135414534399, 0.6588822455111159604, 0.2968425708877995284 ) ) ;
#12573=LINE ( 'NONE', #9441, #6697 ) ;
#12574=DIRECTION ( 'NONE',  ( -1.000000000000000000, 0.000000000000000000, 0.000000000000000000 ) ) ;
#12586=EDGE_CURVE ( 'NONE', #38550, #9701, #23971, .T. ) ;
#12598=CARTESIAN_POINT ( 'NONE',  ( -0.3161444924769509779, 1.209494567139727250, -1.479906699140296045 ) ) ;
#12662=ORIENTED_EDGE ( 'NONE', *, *, #47026, .T. ) ;
#12701=CYLINDRICAL_SURFACE ( 'NONE', #39155, 0.4724409448818896462 ) ;
#12705=ADVANCED_FACE ( 'NONE', ( #20358 ), #34996, .F. ) ;
#12706=VERTEX_POINT ( 'NONE', #34295 ) ;
#12727=DIRECTION ( 'NONE',  ( 0.000000000000000000, 0.000000000000000000, 1.000000000000000000 ) ) ;
#12783=CARTESIAN_POINT ( 'NONE',  ( -0.3161444924769509779, 2.177585298233989164, -3.731703755406937439 ) ) ;
#12809=EDGE_CURVE ( 'NONE', #44905, #15659, #24377, .T. ) ;
#12855=AXIS2_PLACEMENT_3D ( 'NONE', #1037, #18551, #15695 ) ;
#12894=ORIENTED_EDGE ( 'NONE', *, *, #24208, .F. ) ;
#12903=EDGE_CURVE ( 'NONE', #33336, #19054, #39260, .T. ) ;
#12949=LINE ( 'NONE', #31167, #35239 ) ;
#12954=DIRECTION ( 'NONE',  ( 0.6018150231520413840, -0.000000000000000000, -0.7986355100472980473 ) ) ;
#12962=CIRCLE ( 'NONE', #44328, 0.5905511811023623769 ) ;
#13002=ORIENTED_EDGE ( 'NONE', *, *, #22296, .F. ) ;
#13046=DIRECTION ( 'NONE',  ( -1.000000000000000000, 0.000000000000000000, 0.000000000000000000 ) ) ;
#13081=VERTEX_POINT ( 'NONE', #22003 ) ;
#13096=AXIS2_PLACEMENT_3D ( 'NONE', #10448, #6824, #36071 ) ;
#13121=EDGE_CURVE ( 'NONE', #26635, #36995, #41838, .T. ) ;
#13132=VERTEX_POINT ( 'NONE', #16017 ) ;
#13143=ORIENTED_EDGE ( 'NONE', *, *, #36841, .T. ) ;
#13144=EDGE_CURVE ( 'NONE', #47403, #3012, #26568, .T. ) ;
#13163=LINE ( 'NONE', #45232, #22817 ) ;
#13224=ORIENTED_EDGE ( 'NONE', *, *, #14016, .F. ) ;
#13272=DIRECTION ( 'NONE',  ( 1.000000000000000000, -0.000000000000000000, -0.000000000000000000 ) ) ;
#13288=DIRECTION ( 'NONE',  ( 0.000000000000000000, 0.7880107536067203489, -0.6156614753256604011 ) ) ;
#13297=ORIENTED_EDGE ( 'NONE', *, *, #15550, .F. ) ;
#13384=CARTESIAN_POINT ( 'NONE',  ( -0.1586641775163213364, 2.177585298233989164, -3.731703755406937439 ) ) ;
#13388=EDGE_CURVE ( 'NONE', #32649, #40831, #5276, .T. ) ;
#13393=VECTOR ( 'NONE', #11296, 39.37007874015748854 ) ;
#13395=LINE ( 'NONE', #42584, #25346 ) ;
#13421=CARTESIAN_POINT ( 'NONE',  ( -0.1184675242425147629, -0.09842519685039370636, 1.713085361781125471 ) ) ;
#13477=PLANE ( 'NONE',  #18511 ) ;
#13577=DIRECTION ( 'NONE',  ( -1.000000000000000000, 0.000000000000000000, 0.000000000000000000 ) ) ;
#13599=CARTESIAN_POINT ( 'NONE',  ( -0.3161444924769509779, 1.798092712879851174, -3.826876940038414610 ) ) ;
#13604=CARTESIAN_POINT ( 'NONE',  ( -0.08091701073424910351, -0.5708661417322834497, 1.112073044918589382 ) ) ;
#13619=ORIENTED_EDGE ( 'NONE', *, *, #4750, .F. ) ;
#13628=AXIS2_PLACEMENT_3D ( 'NONE', #31505, #42951, #46088 ) ;
#13648=AXIS2_PLACEMENT_3D ( 'NONE', #28975, #46657, #46896 ) ;
#13700=DIRECTION ( 'NONE',  ( 1.000000000000000000, 0.000000000000000000, -0.000000000000000000 ) ) ;
#13737=LINE ( 'NONE', #28379, #43857 ) ;
#13753=ORIENTED_EDGE ( 'NONE', *, *, #40538, .T. ) ;
#13773=CARTESIAN_POINT ( 'NONE',  ( 0.1574803149606299746, 0.4003652867858630282, 0.7276473417831955670 ) ) ;
#13816=EDGE_LOOP ( 'NONE', ( #35048, #13143, #3510, #34672, #35171 ) ) ;
#13818=DIRECTION ( 'NONE',  ( 0.000000000000000000, 0.000000000000000000, -1.000000000000000000 ) ) ;
#13830=DIRECTION ( 'NONE',  ( 0.000000000000000000, 1.000000000000000000, 0.000000000000000000 ) ) ;
#13859=CIRCLE ( 'NONE', #10801, 0.7874015748031437667 ) ;
#13861=ORIENTED_EDGE ( 'NONE', *, *, #1947, .T. ) ;
#13883=ORIENTED_EDGE ( 'NONE', *, *, #26152, .T. ) ;
#13909=EDGE_CURVE ( 'NONE', #47403, #24855, #388, .T. ) ;
#13963=AXIS2_PLACEMENT_3D ( 'NONE', #33731, #15501, #44685 ) ;
#13965=CARTESIAN_POINT ( 'NONE',  ( 0.000000000000000000, -5.122214988120488358E-16, -8.878505979408856939E-16 ) ) ;
#14016=EDGE_CURVE ( 'NONE', #7415, #28468, #20475, .T. ) ;
#14070=DIRECTION ( 'NONE',  ( 0.5735764363510330588, -0.6455006197386629063, 0.5043203561029945270 ) ) ;
#14071=EDGE_CURVE ( 'NONE', #10268, #3060, #9705, .T. ) ;
#14143=ORIENTED_EDGE ( 'NONE', *, *, #23981, .T. ) ;
#14162=VERTEX_POINT ( 'NONE', #21171 ) ;
#14231=DIRECTION ( 'NONE',  ( 0.000000000000000000, 0.000000000000000000, 1.000000000000000000 ) ) ;
#14244=EDGE_LOOP ( 'NONE', ( #5151, #12465, #29384, #45141 ) ) ;
#14329=CARTESIAN_POINT ( 'NONE',  ( 0.03901279071809810040, -0.5708661417322835607, 1.224299699984025658 ) ) ;
#14333=PLANE ( 'NONE',  #10106 ) ;
#14362=CARTESIAN_POINT ( 'NONE',  ( 0.1574803149606339714, 0.9310112235910574796, -1.064878870394357468 ) ) ;
#14363=EDGE_CURVE ( 'NONE', #5917, #19054, #12962, .T. ) ;
#14369=EDGE_LOOP ( 'NONE', ( #16469, #13753, #4040, #4301, #14143, #44564, #23058, #34444, #46094, #37583, #47087, #33184 ) ) ;
#14440=LINE ( 'NONE', #36489, #4593 ) ;
#14479=CARTESIAN_POINT ( 'NONE',  ( -0.3161444924769509779, 1.025704337919491005, -1.138861239548321524 ) ) ;
#14531=VECTOR ( 'NONE', #34559, 39.37007874015748143 ) ;
#14540=ORIENTED_EDGE ( 'NONE', *, *, #35690, .T. ) ;
#14565=ORIENTED_EDGE ( 'NONE', *, *, #26639, .T. ) ;
#14572=FACE_OUTER_BOUND ( 'NONE', #36459, .T. ) ;
#14624=VECTOR ( 'NONE', #30485, 39.37007874015748854 ) ;
#14640=LINE ( 'NONE', #17282, #1493 ) ;
#14696=FACE_OUTER_BOUND ( 'NONE', #14244, .T. ) ;
#14758=DIRECTION ( 'NONE',  ( 1.000000000000000000, -0.000000000000000000, -0.000000000000000000 ) ) ;
#14796=CIRCLE ( 'NONE', #41537, 0.3937007874015748254 ) ;
#14808=DIRECTION ( 'NONE',  ( 1.000000000000000000, -0.000000000000000000, -0.000000000000000000 ) ) ;
#14870=ORIENTED_EDGE ( 'NONE', *, *, #27350, .T. ) ;
#14876=DIRECTION ( 'NONE',  ( 0.000000000000000000, 0.000000000000000000, -1.000000000000000000 ) ) ;
#14897=CIRCLE ( 'NONE', #11848, 0.7874015748031437667 ) ;
#14903=( CONVERSION_BASED_UNIT ( 'INCH', #25920 ) LENGTH_UNIT ( ) NAMED_UNIT ( #16697 ) ) ;
#14910=LINE ( 'NONE', #29572, #3984 ) ;
#14952=DIRECTION ( 'NONE',  ( 0.000000000000000000, 0.000000000000000000, 1.000000000000000000 ) ) ;
#15067=DIRECTION ( 'NONE',  ( 0.000000000000000000, 0.6156614753256575145, 0.7880107536067224583 ) ) ;
#15072=CARTESIAN_POINT ( 'NONE',  ( 0.000000000000000000, 0.6241017553149654784, 0.3240160679609099259 ) ) ;
#15124=EDGE_CURVE ( 'NONE', #22445, #28080, #4125, .T. ) ;
#15128=ORIENTED_EDGE ( 'NONE', *, *, #43493, .F. ) ;
#15141=CYLINDRICAL_SURFACE ( 'NONE', #5658, 0.3912448816427701037 ) ;
#15169=CARTESIAN_POINT ( 'NONE',  ( -0.3161444924769509779, 1.209494567139727250, -1.479906699140296045 ) ) ;
#15189=EDGE_LOOP ( 'NONE', ( #37385, #31133, #31022, #12059 ) ) ;
#15204=SURFACE_SIDE_STYLE ('',( #30322 ) ) ;
#15210=EDGE_CURVE ( 'NONE', #10497, #28468, #45319, .T. ) ;
#15214=DIRECTION ( 'NONE',  ( 1.000000000000000000, -0.000000000000000000, -0.000000000000000000 ) ) ;
#15233=EDGE_CURVE ( 'NONE', #18913, #18496, #45546, .T. ) ;
#15286=VECTOR ( 'NONE', #408, 39.37007874015748143 ) ;
#15453=CIRCLE ( 'NONE', #16948, 0.1864803149606299448 ) ;
#15501=DIRECTION ( 'NONE',  ( -0.000000000000000000, -0.6156614753256605121, -0.7880107536067204599 ) ) ;
#15502=CARTESIAN_POINT ( 'NONE',  ( -0.3161444924769509779, 2.177585298233989164, -3.731703755406937439 ) ) ;
#15522=LINE ( 'NONE', #22691, #28260 ) ;
#15550=EDGE_CURVE ( 'NONE', #33336, #22445, #14640, .T. ) ;
#15557=PRODUCT_DEFINITION_FORMATION_WITH_SPECIFIED_SOURCE ( 'ANY', '', #19185, .NOT_KNOWN. ) ;
#15570=CARTESIAN_POINT ( 'NONE',  ( -0.1184675242425147629, -0.09842519685039370636, 1.870565676741754668 ) ) ;
#15633=CARTESIAN_POINT ( 'NONE',  ( 0.000000000000000000, 0.3883517482604934012, -0.6419475548153109612 ) ) ;
#15659=VERTEX_POINT ( 'NONE', #34057 ) ;
#15695=DIRECTION ( 'NONE',  ( 0.000000000000000000, 0.000000000000000000, -1.000000000000000000 ) ) ;
#15786=CARTESIAN_POINT ( 'NONE',  ( -0.1534195868007020847, 0.9251089822459547252, -1.060267534067255157 ) ) ;
#15820=EDGE_CURVE ( 'NONE', #32649, #40086, #12949, .T. ) ;
#15829=CARTESIAN_POINT ( 'NONE',  ( -0.02900000000000056352, 0.5288907983920048128, -0.7507079620615672022 ) ) ;
#15923=ORIENTED_EDGE ( 'NONE', *, *, #4801, .T. ) ;
#15967=EDGE_LOOP ( 'NONE', ( #35114, #36362, #17529, #28807 ) ) ;
#15979=CARTESIAN_POINT ( 'NONE',  ( 0.000000000000000000, -0.5708661417322835607, 0.9783464566929281903 ) ) ;
#16017=CARTESIAN_POINT ( 'NONE',  ( -0.2824199087359778315, 0.8539303365987040983, -1.004656681308842225 ) ) ;
#16045=CARTESIAN_POINT ( 'NONE',  ( 0.1574803149606299746, 0.1473293504822046074, -0.9532488779249699284 ) ) ;
#16064=ORIENTED_EDGE ( 'NONE', *, *, #33421, .F. ) ;
#16129=ORIENTED_EDGE ( 'NONE', *, *, #10122, .F. ) ;
#16180=DIRECTION ( 'NONE',  ( -1.000000000000000000, 0.000000000000000000, 0.000000000000000000 ) ) ;
#16236=EDGE_CURVE ( 'NONE', #3991, #3105, #44488, .T. ) ;
#16284=ORIENTED_EDGE ( 'NONE', *, *, #43207, .T. ) ;
#16335=VECTOR ( 'NONE', #5464, 39.37007874015748143 ) ;
#16377=EDGE_CURVE ( 'NONE', #17177, #22261, #34697, .T. ) ;
#16469=ORIENTED_EDGE ( 'NONE', *, *, #23438, .F. ) ;
#16587=DIRECTION ( 'NONE',  ( 0.6018150231520356108, -0.000000000000000000, -0.7986355100473022661 ) ) ;
#16642=PLANE ( 'NONE',  #13628 ) ;
#16648=VERTEX_POINT ( 'NONE', #26990 ) ;
#16697=DIMENSIONAL_EXPONENTS ( 1.000000000000000000, 0.000000000000000000, 0.000000000000000000, 0.000000000000000000, 0.000000000000000000, 0.000000000000000000, 0.000000000000000000 ) ;
#16714=FACE_OUTER_BOUND ( 'NONE', #533, .T. ) ;
#16756=EDGE_LOOP ( 'NONE', ( #20238, #13861, #20365, #22271 ) ) ;
#16875=AXIS2_PLACEMENT_3D ( 'NONE', #43061, #10265, #26312 ) ;
#16947=VECTOR ( 'NONE', #18686, 39.37007874015748143 ) ;
#16948=AXIS2_PLACEMENT_3D ( 'NONE', #31307, #30847, #2044 ) ;
#16971=DIRECTION ( 'NONE',  ( 0.000000000000000000, 0.000000000000000000, -1.000000000000000000 ) ) ;
#16978=DIRECTION ( 'NONE',  ( 0.000000000000000000, 0.6156614753256639538, 0.7880107536067174623 ) ) ;
#16993=DIRECTION ( 'NONE',  ( 0.000000000000000000, -0.7880107536067201268, 0.6156614753256606232 ) ) ;
#17097=DIRECTION ( 'NONE',  ( 0.000000000000000000, 0.000000000000000000, 1.000000000000000000 ) ) ;
#17177=VERTEX_POINT ( 'NONE', #29595 ) ;
#17188=DIRECTION ( 'NONE',  ( 0.000000000000000000, 0.000000000000000000, -1.000000000000000000 ) ) ;
#17264=ADVANCED_FACE ( 'NONE', ( #11335 ), #7480, .F. ) ;
#17282=CARTESIAN_POINT ( 'NONE',  ( 0.1574803149606299746, 0.3740157480314960647, 0.9783464566929134243 ) ) ;
#17342=ORIENTED_EDGE ( 'NONE', *, *, #29606, .T. ) ;
#17354=EDGE_LOOP ( 'NONE', ( #20613, #7567, #39217, #45326 ) ) ;
#17359=ORIENTED_EDGE ( 'NONE', *, *, #33751, .F. ) ;
#17436=DIRECTION ( 'NONE',  ( -1.000000000000000000, 0.000000000000000000, 0.000000000000000000 ) ) ;
#17438=CARTESIAN_POINT ( 'NONE',  ( 0.03901279071809810040, 0.3740157480314960647, 1.057384721142220263 ) ) ;
#17440=FACE_OUTER_BOUND ( 'NONE', #126, .T. ) ;
#17462=CARTESIAN_POINT ( 'NONE',  ( -0.1586641775163213364, 2.177585298233989164, -3.731703755406937439 ) ) ;
#17475=CARTESIAN_POINT ( 'NONE',  ( -0.1184675242425147629, -0.5708661417322835607, 1.713085361781126803 ) ) ;
#17529=ORIENTED_EDGE ( 'NONE', *, *, #3692, .F. ) ;
#17607=DIRECTION ( 'NONE',  ( 0.000000000000000000, -8.240357684727058740E-16, 1.000000000000000000 ) ) ;
#17630=ORIENTED_EDGE ( 'NONE', *, *, #24843, .T. ) ;
#17672=DIRECTION ( 'NONE',  ( 0.000000000000000000, 0.000000000000000000, 1.000000000000000000 ) ) ;
#17673=ORIENTED_EDGE ( 'NONE', *, *, #27123, .T. ) ;
#17696=EDGE_CURVE ( 'NONE', #15659, #46267, #22790, .T. ) ;
#17703=LINE ( 'NONE', #10777, #4984 ) ;
#17740=EDGE_LOOP ( 'NONE', ( #10872, #31700, #5131, #35749 ) ) ;
#17831=ORIENTED_EDGE ( 'NONE', *, *, #23981, .F. ) ;
#17844=EDGE_CURVE ( 'NONE', #5685, #4833, #39986, .T. ) ;
#17847=FACE_OUTER_BOUND ( 'NONE', #36870, .T. ) ;
#17852=COLOUR_RGB ( '', 0.72549020, 0.75294118, 0.79215686) ;
#17894=ORIENTED_EDGE ( 'NONE', *, *, #18187, .F. ) ;
#17895=FACE_OUTER_BOUND ( 'NONE', #5252, .T. ) ;
#17995=ORIENTED_EDGE ( 'NONE', *, *, #47026, .F. ) ;
#18015=EDGE_CURVE ( 'NONE', #18496, #33336, #46006, .T. ) ;
#18067=CARTESIAN_POINT ( 'NONE',  ( -0.01585547164981878157, 0.3740157480314960647, 1.025733466389939785 ) ) ;
#18068=CARTESIAN_POINT ( 'NONE',  ( 0.000000000000000000, 3.616083068348478250E-17, 0.2952755905511806334 ) ) ;
#18109=DIRECTION ( 'NONE',  ( 0.000000000000000000, 0.000000000000000000, -1.000000000000000000 ) ) ;
#18187=EDGE_CURVE ( 'NONE', #23245, #45939, #45975, .T. ) ;
#18233=ORIENTED_EDGE ( 'NONE', *, *, #27301, .T. ) ;
#18372=ORIENTED_EDGE ( 'NONE', *, *, #36382, .F. ) ;
#18385=VERTEX_POINT ( 'NONE', #5467 ) ;
#18393=ADVANCED_FACE ( 'NONE', ( #24394 ), #20082, .T. ) ;
#18402=ORIENTED_EDGE ( 'NONE', *, *, #18930, .T. ) ;
#18434=CARTESIAN_POINT ( 'NONE',  ( 0.1574803149606300023, 3.616083068348478250E-17, 0.2952755905511806334 ) ) ;
#18470=LINE ( 'NONE', #40022, #13393 ) ;
#18496=VERTEX_POINT ( 'NONE', #6400 ) ;
#18511=AXIS2_PLACEMENT_3D ( 'NONE', #12783, #13700, #20648 ) ;
#18530=ORIENTED_EDGE ( 'NONE', *, *, #36916, .T. ) ;
#18551=DIRECTION ( 'NONE',  ( -1.000000000000000000, 0.000000000000000000, 0.000000000000000000 ) ) ;
#18583=DIRECTION ( 'NONE',  ( 0.000000000000000000, 0.000000000000000000, -1.000000000000000000 ) ) ;
#18686=DIRECTION ( 'NONE',  ( -1.000000000000000000, 0.000000000000000000, -0.000000000000000000 ) ) ;
#18708=( NAMED_UNIT ( * ) SI_UNIT ( $, .STERADIAN. ) SOLID_ANGLE_UNIT ( ) ) ;
#18723=CARTESIAN_POINT ( 'NONE',  ( 0.000000000000000000, 0.000000000000000000, -0.2952755905511806334 ) ) ;
#18778=( LENGTH_UNIT ( ) NAMED_UNIT ( * ) SI_UNIT ( $, .METRE. ) ) ;
#18796=VERTEX_POINT ( 'NONE', #11206 ) ;
#18804=DIRECTION ( 'NONE',  ( 0.000000000000000000, 0.000000000000000000, 1.000000000000000000 ) ) ;
#18913=VERTEX_POINT ( 'NONE', #30604 ) ;
#18930=EDGE_CURVE ( 'NONE', #39413, #10497, #15453, .T. ) ;
#18993=LINE ( 'NONE', #14479, #27764 ) ;
#19054=VERTEX_POINT ( 'NONE', #13773 ) ;
#19092=CIRCLE ( 'NONE', #43580, 0.2952755905511806334 ) ;
#19139=ORIENTED_EDGE ( 'NONE', *, *, #10512, .T. ) ;
#19185=PRODUCT ( 'Handle Arm Left', 'Handle Arm Left', '', ( #27426 ) ) ;
#19229=VECTOR ( 'NONE', #44062, 39.37007874015748854 ) ;
#19259=ORIENTED_EDGE ( 'NONE', *, *, #13388, .F. ) ;
#19271=ORIENTED_EDGE ( 'NONE', *, *, #31516, .F. ) ;
#19281=UNCERTAINTY_MEASURE_WITH_UNIT (LENGTH_MEASURE( 1.000000000000000082E-05 ), #14903, 'distance_accuracy_value', 'NONE') ;
#19425=DIRECTION ( 'NONE',  ( 0.000000000000000000, 2.602085213965210247E-15, -1.000000000000000000 ) ) ;
#19432=DIRECTION ( 'NONE',  ( -8.673617379884043361E-16, 0.000000000000000000, -1.000000000000000000 ) ) ;
#19449=CARTESIAN_POINT ( 'NONE',  ( -0.005244590715618953347, 0.5419983459879460508, -0.7609487005970287932 ) ) ;
#19568=CYLINDRICAL_SURFACE ( 'NONE', #38195, 0.02900000000000060515 ) ;
#19630=DIRECTION ( 'NONE',  ( 3.547931780924148305E-15, -0.7880107536067215701, 0.6156614753256588468 ) ) ;
#19633=EDGE_LOOP ( 'NONE', ( #40007, #47346, #40923, #47015 ) ) ;
#19643=EDGE_CURVE ( 'NONE', #41828, #23265, #38661, .T. ) ;
#19710=ORIENTED_EDGE ( 'NONE', *, *, #2710, .F. ) ;
#19762=EDGE_LOOP ( 'NONE', ( #41004, #33807, #26365, #16129 ) ) ;
#19766=EDGE_CURVE ( 'NONE', #33336, #4491, #29982, .T. ) ;
#19826=CARTESIAN_POINT ( 'NONE',  ( -0.3161444924769509779, 2.177585298233989164, -3.731703755406937439 ) ) ;
#19835=AXIS2_PLACEMENT_3D ( 'NONE', #7706, #7001, #36949 ) ;
#19860=ADVANCED_FACE ( 'NONE', ( #44764 ), #9324, .T. ) ;
#19880=CIRCLE ( 'NONE', #1488, 0.1864803149606299171 ) ;
#19885=DIRECTION ( 'NONE',  ( 0.000000000000000000, -0.000000000000000000, -1.000000000000000000 ) ) ;
#19981=CIRCLE ( 'NONE', #13096, 0.1864803149606300003 ) ;
#20072=ADVANCED_FACE ( 'NONE', ( #17440 ), #28490, .T. ) ;
#20080=VECTOR ( 'NONE', #13046, 39.37007874015748143 ) ;
#20082=PLANE ( 'NONE',  #32298 ) ;
#20147=DIRECTION ( 'NONE',  ( -0.000000000000000000, -0.7880107536067176843, 0.6156614753256636208 ) ) ;
#20173=CARTESIAN_POINT ( 'NONE',  ( 0.1574803149606299746, 0.6241017553149654784, 0.3240160679609099259 ) ) ;
#20206=CARTESIAN_POINT ( 'NONE',  ( 0.1574803149606299746, 0.3740157480314960647, 1.713085361781126803 ) ) ;
#20236=DIRECTION ( 'NONE',  ( 0.000000000000000000, 0.6156614753256575145, 0.7880107536067225693 ) ) ;
#20238=ORIENTED_EDGE ( 'NONE', *, *, #47358, .F. ) ;
#20326=FACE_OUTER_BOUND ( 'NONE', #16756, .T. ) ;
#20358=FACE_OUTER_BOUND ( 'NONE', #37718, .T. ) ;
#20365=ORIENTED_EDGE ( 'NONE', *, *, #38804, .T. ) ;
#20475=LINE ( 'NONE', #46104, #38967 ) ;
#20530=CIRCLE ( 'NONE', #13648, 0.3912448816427701037 ) ;
#20566=EDGE_CURVE ( 'NONE', #3060, #42269, #19981, .T. ) ;
#20600=CARTESIAN_POINT ( 'NONE',  ( -0.1586641775163213364, 2.559880088878760951, -3.648497683167374550 ) ) ;
#20613=ORIENTED_EDGE ( 'NONE', *, *, #20566, .F. ) ;
#20648=DIRECTION ( 'NONE',  ( -0.000000000000000000, 0.000000000000000000, -1.000000000000000000 ) ) ;
#20690=CARTESIAN_POINT ( 'NONE',  ( -0.1184675242425147906, -0.09842519685039370636, 1.713085361781125471 ) ) ;
#20763=CARTESIAN_POINT ( 'NONE',  ( 0.1237557312196567866, 1.170665729134807931, -0.1030065087509293015 ) ) ;
#20794=DIRECTION ( 'NONE',  ( 0.000000000000000000, 0.000000000000000000, 1.000000000000000000 ) ) ;
#20828=ORIENTED_EDGE ( 'NONE', *, *, #43207, .F. ) ;
#20849=ORIENTED_EDGE ( 'NONE', *, *, #40550, .F. ) ;
#20860=AXIS2_PLACEMENT_3D ( 'NONE', #25692, #32652, #10835 ) ;
#20883=DIRECTION ( 'NONE',  ( -1.000000000000000000, 0.000000000000000000, 0.000000000000000000 ) ) ;
#20925=CARTESIAN_POINT ( 'NONE',  ( -0.1184675242425147629, 0.3740157480314960647, 1.224299699984020551 ) ) ;
#21003=CARTESIAN_POINT ( 'NONE',  ( -0.1586641775163213364, 0.9310112235910577017, -1.064878870394357691 ) ) ;
#21052=DIRECTION ( 'NONE',  ( 0.000000000000000000, 0.1045284632676499320, -0.9945218953682736229 ) ) ;
#21061=AXIS2_PLACEMENT_3D ( 'NONE', #10117, #24728, #46758 ) ;
#21076=DIRECTION ( 'NONE',  ( 0.000000000000000000, 0.000000000000000000, 1.000000000000000000 ) ) ;
#21088=LINE ( 'NONE', #10573, #37455 ) ;
#21137=DIRECTION ( 'NONE',  ( 0.7986355100472981583, -0.000000000000000000, 0.6018150231520413840 ) ) ;
#21164=ORIENTED_EDGE ( 'NONE', *, *, #24208, .T. ) ;
#21171=CARTESIAN_POINT ( 'NONE',  ( 0.03901279071809810040, -0.09842519685039370636, 2.185526306663017504 ) ) ;
#21246=FACE_OUTER_BOUND ( 'NONE', #31862, .T. ) ;
#21260=FACE_OUTER_BOUND ( 'NONE', #15967, .T. ) ;
#21261=DIRECTION ( 'NONE',  ( 1.000000000000000000, 0.000000000000000000, 0.000000000000000000 ) ) ;
#21311=CARTESIAN_POINT ( 'NONE',  ( -0.1184675242425147629, -0.09842519685039327615, 1.224299699984020107 ) ) ;
#21312=DIRECTION ( 'NONE',  ( 1.766281030386342844E-15, 0.000000000000000000, -1.000000000000000000 ) ) ;
#21351=DIRECTION ( 'NONE',  ( 1.000000000000000000, -0.000000000000000000, -0.000000000000000000 ) ) ;
#21354=EDGE_CURVE ( 'NONE', #37269, #23265, #3377, .T. ) ;
#21427=DIRECTION ( 'NONE',  ( -1.363218471095259303E-17, -0.6156614753256575145, -0.7880107536067225693 ) ) ;
#21465=DIRECTION ( 'NONE',  ( -1.177520686924230272E-15, -0.7880107536067199048, 0.6156614753256609562 ) ) ;
#21476=AXIS2_PLACEMENT_3D ( 'NONE', #24178, #2340, #16971 ) ;
#21582=VECTOR ( 'NONE', #32122, 39.37007874015748143 ) ;
#21596=DIRECTION ( 'NONE',  ( 1.000000000000000000, -0.000000000000000000, -0.000000000000000000 ) ) ;
#21637=ORIENTED_EDGE ( 'NONE', *, *, #42977, .T. ) ;
#21657=ADVANCED_FACE ( 'NONE', ( #43534, #47149 ), #14333, .F. ) ;
#21755=EDGE_LOOP ( 'NONE', ( #42662, #28128, #44270, #7087 ) ) ;
#21781=DIRECTION ( 'NONE',  ( -0.000000000000000000, -0.7880107536067214591, 0.6156614753256588468 ) ) ;
#21805=CARTESIAN_POINT ( 'NONE',  ( -0.1534195868007021402, 0.9251089822459552803, -1.060267534067254935 ) ) ;
#21852=PRODUCT_DEFINITION_SHAPE ( 'NONE', 'NONE',  #754 ) ;
#21866=EDGE_CURVE ( 'NONE', #43609, #18913, #28494, .T. ) ;
#21880=ORIENTED_EDGE ( 'NONE', *, *, #42977, .F. ) ;
#21955=CYLINDRICAL_SURFACE ( 'NONE', #11137, 0.02900000000000056352 ) ;
#22003=CARTESIAN_POINT ( 'NONE',  ( 0.000000000000000000, 1.086379535891621506, -0.03715491745705968435 ) ) ;
#22030=CIRCLE ( 'NONE', #43539, 0.1864803149606299171 ) ;
#22036=DIRECTION ( 'NONE',  ( 0.000000000000000000, -0.1045284632676499320, 0.9945218953682736229 ) ) ;
#22065=ORIENTED_EDGE ( 'NONE', *, *, #16377, .F. ) ;
#22070=CIRCLE ( 'NONE', #29754, 0.1864803149606298893 ) ;
#22233=VECTOR ( 'NONE', #35075, 39.37007874015748143 ) ;
#22261=VERTEX_POINT ( 'NONE', #37963 ) ;
#22271=ORIENTED_EDGE ( 'NONE', *, *, #1994, .T. ) ;
#22296=EDGE_CURVE ( 'NONE', #12706, #39516, #34150, .T. ) ;
#22412=VECTOR ( 'NONE', #5710, 39.37007874015747433 ) ;
#22424=CARTESIAN_POINT ( 'NONE',  ( 0.03901279071809810040, -0.5708661417322835607, 1.713085361781127913 ) ) ;
#22430=DIRECTION ( 'NONE',  ( 1.000000000000000000, -0.000000000000000000, -0.000000000000000000 ) ) ;
#22445=VERTEX_POINT ( 'NONE', #2463 ) ;
#22546=CARTESIAN_POINT ( 'NONE',  ( -0.3161444924769509779, 2.177585298233989164, -3.731703755406937439 ) ) ;
#22650=CARTESIAN_POINT ( 'NONE',  ( -0.08091701073424910351, -0.5708661417322835607, 1.112073044918589382 ) ) ;
#22691=CARTESIAN_POINT ( 'NONE',  ( -0.3161444924769509779, 2.559880088878760951, -3.648497683167374550 ) ) ;
#22736=DIRECTION ( 'NONE',  ( 0.000000000000000000, 0.000000000000000000, 1.000000000000000000 ) ) ;
#22785=SHAPE_REPRESENTATION_RELATIONSHIP ( 'NONE' , 'NONE' ,  #43589, #7828 ) ;
#22790=LINE ( 'NONE', #33844, #14624 ) ;
#22795=CARTESIAN_POINT ( 'NONE',  ( -0.1184675242425147629, 0.3740157480314960647, 1.713085361781126803 ) ) ;
#22807=DIRECTION ( 'NONE',  ( 0.000000000000000000, -0.2432573283306819767, 0.9699617890481142535 ) ) ;
#22817=VECTOR ( 'NONE', #27797, 39.37007874015748854 ) ;
#22818=DIRECTION ( 'NONE',  ( 0.000000000000000000, 0.1045284632676499320, -0.9945218953682736229 ) ) ;
#22881=CARTESIAN_POINT ( 'NONE',  ( 0.1574803149606299746, -0.09842519685039370636, 1.713085361781126803 ) ) ;
#22896=FACE_OUTER_BOUND ( 'NONE', #34458, .T. ) ;
#22904=LINE ( 'NONE', #4916, #37595 ) ;
#22928=FACE_OUTER_BOUND ( 'NONE', #42544, .T. ) ;
#23058=ORIENTED_EDGE ( 'NONE', *, *, #24381, .F. ) ;
#23070=EDGE_CURVE ( 'NONE', #8749, #46267, #24746, .T. ) ;
#23073=CARTESIAN_POINT ( 'NONE',  ( 0.1574803149606299746, 0.3740157480314960647, 0.9783464566929134243 ) ) ;
#23128=ORIENTED_EDGE ( 'NONE', *, *, #19766, .T. ) ;
#23151=CARTESIAN_POINT ( 'NONE',  ( -0.1184675242425147629, 0.3740157480314960647, 1.161904259418922836 ) ) ;
#23172=DIRECTION ( 'NONE',  ( 0.000000000000000000, 0.7880107536067175733, -0.6156614753256638428 ) ) ;
#23186=ORIENTED_EDGE ( 'NONE', *, *, #35719, .F. ) ;
#23206=VECTOR ( 'NONE', #38131, 39.37007874015748143 ) ;
#23243=DIRECTION ( 'NONE',  ( -1.217491584052838080E-15, -0.6156614753256588468, -0.7880107536067214591 ) ) ;
#23245=VERTEX_POINT ( 'NONE', #18723 ) ;
#23249=CARTESIAN_POINT ( 'NONE',  ( 0.03901279071809810040, -0.09842519685039370636, 1.713085361781127913 ) ) ;
#23265=VERTEX_POINT ( 'NONE', #12459 ) ;
#23317=AXIS2_PLACEMENT_3D ( 'NONE', #20690, #10398, #17097 ) ;
#23348=DIRECTION ( 'NONE',  ( 0.000000000000000000, -0.6156614753256639538, -0.7880107536067174623 ) ) ;
#23406=DIRECTION ( 'NONE',  ( -0.000000000000000000, -0.7880107536067176843, 0.6156614753256636208 ) ) ;
#23435=DIRECTION ( 'NONE',  ( 0.000000000000000000, 0.6156614753256604011, 0.7880107536067203489 ) ) ;
#23438=EDGE_CURVE ( 'NONE', #13132, #35281, #31142, .T. ) ;
#23446=VECTOR ( 'NONE', #21781, 39.37007874015748143 ) ;
#23473=ORIENTED_EDGE ( 'NONE', *, *, #27350, .F. ) ;
#23522=CARTESIAN_POINT ( 'NONE',  ( -0.07874015748031495954, -0.5708661417322835607, 0.9783464566929284123 ) ) ;
#23576=FACE_OUTER_BOUND ( 'NONE', #17740, .T. ) ;
#23709=EDGE_CURVE ( 'NONE', #5685, #37269, #43814, .T. ) ;
#23729=CARTESIAN_POINT ( 'NONE',  ( 0.1574803149606299746, -0.5708661417322835607, -6.991093932140394160E-17 ) ) ;
#23905=VECTOR ( 'NONE', #11209, 39.37007874015748854 ) ;
#23929=CARTESIAN_POINT ( 'NONE',  ( 0.03901279071809810040, -0.09842519685039369248, 1.555605046820496273 ) ) ;
#23945=CARTESIAN_POINT ( 'NONE',  ( -0.07874015748031489015, -0.5708661417322835607, 0.9783464566929127582 ) ) ;
#23971=LINE ( 'NONE', #34061, #5242 ) ;
#23980=VERTEX_POINT ( 'NONE', #27617 ) ;
#23981=EDGE_CURVE ( 'NONE', #33937, #30045, #45057, .T. ) ;
#24085=VECTOR ( 'NONE', #28530, 39.37007874015748854 ) ;
#24136=CIRCLE ( 'NONE', #30278, 0.4724409448818896462 ) ;
#24175=FACE_OUTER_BOUND ( 'NONE', #14369, .T. ) ;
#24178=CARTESIAN_POINT ( 'NONE',  ( 0.1574803149606299746, 0.000000000000000000, 0.000000000000000000 ) ) ;
#24208=EDGE_CURVE ( 'NONE', #36995, #42269, #30732, .T. ) ;
#24310=ADVANCED_FACE ( 'NONE', ( #40891 ), #8084, .T. ) ;
#24318=CARTESIAN_POINT ( 'NONE',  ( 0.05249343832021334533, 0.4668427075568369333, -0.7022306805398672580 ) ) ;
#24339=CARTESIAN_POINT ( 'NONE',  ( 0.1574803149606299746, 0.4666052258408023845, -0.7025346432751043979 ) ) ;
#24363=ORIENTED_EDGE ( 'NONE', *, *, #35719, .T. ) ;
#24377=CIRCLE ( 'NONE', #9088, 0.3912448816427701037 ) ;
#24381=EDGE_CURVE ( 'NONE', #28928, #26635, #12173, .T. ) ;
#24394=FACE_OUTER_BOUND ( 'NONE', #6595, .T. ) ;
#24483=AXIS2_PLACEMENT_3D ( 'NONE', #25790, #14758, #18109 ) ;
#24494=FACE_OUTER_BOUND ( 'NONE', #33587, .T. ) ;
#24556=DIRECTION ( 'NONE',  ( 0.000000000000000000, 0.000000000000000000, 1.000000000000000000 ) ) ;
#24566=FACE_OUTER_BOUND ( 'NONE', #44136, .T. ) ;
#24602=ORIENTED_EDGE ( 'NONE', *, *, #26648, .T. ) ;
#24632=CIRCLE ( 'NONE', #122, 0.3937007874015748254 ) ;
#24677=EDGE_CURVE ( 'NONE', #23265, #18385, #44617, .T. ) ;
#24712=AXIS2_PLACEMENT_3D ( 'NONE', #38776, #10501, #5935 ) ;
#24728=DIRECTION ( 'NONE',  ( 1.000000000000000000, -0.000000000000000000, -0.000000000000000000 ) ) ;
#24731=AXIS2_PLACEMENT_3D ( 'NONE', #4012, #15067, #33291 ) ;
#24746=LINE ( 'NONE', #42926, #37670 ) ;
#24843=EDGE_CURVE ( 'NONE', #18796, #6378, #14796, .T. ) ;
#24855=VERTEX_POINT ( 'NONE', #6924 ) ;
#24857=CARTESIAN_POINT ( 'NONE',  ( 0.000000000000000000, 0.4666052258408023845, -0.7025346432751043979 ) ) ;
#24910=VECTOR ( 'NONE', #38042, 39.37007874015748854 ) ;
#24944=AXIS2_PLACEMENT_3D ( 'NONE', #43288, #32054, #6391 ) ;
#24976=CARTESIAN_POINT ( 'NONE',  ( 0.1574803149606299746, 0.08719492171395765157, -0.5641677032617172793 ) ) ;
#25115=DIRECTION ( 'NONE',  ( -0.6018150231520356108, -6.927058840138832622E-16, 0.7986355100473022661 ) ) ;
#25222=VERTEX_POINT ( 'NONE', #36879 ) ;
#25346=VECTOR ( 'NONE', #46664, 39.37007874015748143 ) ;
#25426=DIRECTION ( 'NONE',  ( -0.000000000000000000, 0.7880107536067174623, -0.6156614753256640649 ) ) ;
#25429=ORIENTED_EDGE ( 'NONE', *, *, #44807, .T. ) ;
#25470=CARTESIAN_POINT ( 'NONE',  ( 0.000000000000000000, -1.360801781844024705E-15, 0.9783464566929289674 ) ) ;
#25515=STYLED_ITEM ( 'NONE', ( #4152 ), #36032 ) ;
#25526=EDGE_CURVE ( 'NONE', #24855, #39709, #3029, .T. ) ;
#25599=CARTESIAN_POINT ( 'NONE',  ( 0.1574803149606299746, -5.122214988120488358E-16, -8.878505979408856939E-16 ) ) ;
#25617=EDGE_CURVE ( 'NONE', #14162, #3991, #11033, .T. ) ;
#25662=ORIENTED_EDGE ( 'NONE', *, *, #38469, .F. ) ;
#25692=CARTESIAN_POINT ( 'NONE',  ( 0.000000000000000000, 0.000000000000000000, 0.000000000000000000 ) ) ;
#25712=AXIS2_PLACEMENT_3D ( 'NONE', #6861, #39214, #545 ) ;
#25715=ORIENTED_EDGE ( 'NONE', *, *, #14363, .F. ) ;
#25790=CARTESIAN_POINT ( 'NONE',  ( 0.1574803149606300023, 0.000000000000000000, 0.000000000000000000 ) ) ;
#25875=VECTOR ( 'NONE', #7410, 39.37007874015748143 ) ;
#25909=EDGE_LOOP ( 'NONE', ( #17342, #27808, #36724, #5016, #10522, #3602, #29707, #47046, #17673, #616, #12894, #10278 ) ) ;
#25919=DIRECTION ( 'NONE',  ( 0.000000000000000000, 0.000000000000000000, -1.000000000000000000 ) ) ;
#25920=LENGTH_MEASURE_WITH_UNIT ( LENGTH_MEASURE( 0.02539999999999999897 ), #43876 ) ;
#25948=AXIS2_PLACEMENT_3D ( 'NONE', #24339, #41807, #9725 ) ;
#25984=LINE ( 'NONE', #40566, #30986 ) ;
#26044=CIRCLE ( 'NONE', #27587, 0.07874015748031489015 ) ;
#26061=EDGE_LOOP ( 'NONE', ( #9198, #23128, #9707, #6201, #17630, #4518, #45374, #11786, #34566, #31801, #8038 ) ) ;
#26093=ADVANCED_FACE ( 'NONE', ( #36998, #39626 ), #29631, .F. ) ;
#26152=EDGE_CURVE ( 'NONE', #42269, #28928, #25984, .T. ) ;
#26154=ORIENTED_EDGE ( 'NONE', *, *, #2644, .T. ) ;
#26165=( NAMED_UNIT ( * ) PLANE_ANGLE_UNIT ( ) SI_UNIT ( $, .RADIAN. ) ) ;
#26230=ORIENTED_EDGE ( 'NONE', *, *, #18187, .T. ) ;
#26312=DIRECTION ( 'NONE',  ( -0.000000000000000000, 0.000000000000000000, -1.000000000000000000 ) ) ;
#26319=ORIENTED_EDGE ( 'NONE', *, *, #17844, .T. ) ;
#26363=ORIENTED_EDGE ( 'NONE', *, *, #30093, .F. ) ;
#26365=ORIENTED_EDGE ( 'NONE', *, *, #18015, .F. ) ;
#26397=VERTEX_POINT ( 'NONE', #30785 ) ;
#26456=AXIS2_PLACEMENT_3D ( 'NONE', #29986, #29749, #11500 ) ;
#26476=CARTESIAN_POINT ( 'NONE',  ( -0.1296641775163210608, 0.9382165298418947419, -1.070508272602715083 ) ) ;
#26486=ORIENTED_EDGE ( 'NONE', *, *, #405, .T. ) ;
#26498=FACE_OUTER_BOUND ( 'NONE', #6123, .T. ) ;
#26568=LINE ( 'NONE', #26799, #44286 ) ;
#26594=ORIENTED_EDGE ( 'NONE', *, *, #39799, .F. ) ;
#26607=LINE ( 'NONE', #41639, #1309 ) ;
#26635=VERTEX_POINT ( 'NONE', #21805 ) ;
#26639=EDGE_CURVE ( 'NONE', #43013, #25222, #4920, .T. ) ;
#26648=EDGE_CURVE ( 'NONE', #38550, #3105, #31735, .T. ) ;
#26675=EDGE_LOOP ( 'NONE', ( #2248, #38816, #39887, #3367 ) ) ;
#26706=FILL_AREA_STYLE_COLOUR ( '', #17852 ) ;
#26715=DIRECTION ( 'NONE',  ( -1.217491584052838080E-15, -0.6156614753256588468, -0.7880107536067214591 ) ) ;
#26749=EDGE_LOOP ( 'NONE', ( #28447, #29047, #38146, #42653 ) ) ;
#26787=EDGE_CURVE ( 'NONE', #6378, #43013, #11976, .T. ) ;
#26797=CARTESIAN_POINT ( 'NONE',  ( -0.1586641775163213364, 0.9310112235910580347, -1.064878870394357468 ) ) ;
#26799=CARTESIAN_POINT ( 'NONE',  ( 0.1574803149606299746, 0.4666052258408023845, -0.7025346432751043979 ) ) ;
#26824=DIRECTION ( 'NONE',  ( -1.000000000000000000, -0.000000000000000000, -0.000000000000000000 ) ) ;
#26868=FACE_OUTER_BOUND ( 'NONE', #44989, .T. ) ;
#26947=APPLICATION_CONTEXT ( 'automotive_design' ) ;
#26954=CARTESIAN_POINT ( 'NONE',  ( 0.000000000000000000, 0.4003652867858630282, 0.7276473417831955670 ) ) ;
#26990=CARTESIAN_POINT ( 'NONE',  ( -0.1184675242425147629, -0.5708661417322835607, 1.713085361781126803 ) ) ;
#27075=DIRECTION ( 'NONE',  ( 1.217491584052838080E-15, 0.6156614753256588468, 0.7880107536067214591 ) ) ;
#27116=PLANE ( 'NONE',  #5988 ) ;
#27123=EDGE_CURVE ( 'NONE', #5917, #3060, #13163, .T. ) ;
#27301=EDGE_CURVE ( 'NONE', #18385, #5685, #6877, .T. ) ;
#27303=CARTESIAN_POINT ( 'NONE',  ( -0.3161444924769509779, 0.9382165298418940758, -1.070508272602715749 ) ) ;
#27350=EDGE_CURVE ( 'NONE', #36971, #3855, #20530, .T. ) ;
#27426=PRODUCT_CONTEXT ( 'NONE', #42846, 'mechanical' ) ;
#27537=EDGE_LOOP ( 'NONE', ( #15128, #19259 ) ) ;
#27587=AXIS2_PLACEMENT_3D ( 'NONE', #3302, #32803, #43313 ) ;
#27617=CARTESIAN_POINT ( 'NONE',  ( -0.005244590715618953347, 1.099487083487562522, -0.04739565599252126837 ) ) ;
#27689=ORIENTED_EDGE ( 'NONE', *, *, #47327, .T. ) ;
#27749=AXIS2_PLACEMENT_3D ( 'NONE', #46711, #2392, #43592 ) ;
#27751=CARTESIAN_POINT ( 'NONE',  ( 0.1574803149606299746, 0.000000000000000000, -0.2952755905511806334 ) ) ;
#27754=VECTOR ( 'NONE', #36136, 39.37007874015748143 ) ;
#27764=VECTOR ( 'NONE', #535, 39.37007874015748143 ) ;
#27793=EDGE_CURVE ( 'NONE', #7162, #46787, #1330, .T. ) ;
#27797=DIRECTION ( 'NONE',  ( 0.000000000000000000, 0.7880107536067203489, -0.6156614753256604011 ) ) ;
#27802=FACE_OUTER_BOUND ( 'NONE', #26675, .T. ) ;
#27808=ORIENTED_EDGE ( 'NONE', *, *, #21354, .T. ) ;
#27930=ORIENTED_EDGE ( 'NONE', *, *, #27793, .T. ) ;
#27943=AXIS2_PLACEMENT_3D ( 'NONE', #15502, #41320, #40620 ) ;
#27954=ADVANCED_FACE ( 'NONE', ( #17847 ), #28181, .T. ) ;
#28023=ORIENTED_EDGE ( 'NONE', *, *, #15233, .T. ) ;
#28080=VERTEX_POINT ( 'NONE', #28420 ) ;
#28128=ORIENTED_EDGE ( 'NONE', *, *, #23070, .F. ) ;
#28181=CYLINDRICAL_SURFACE ( 'NONE', #11370, 0.1864803149606298061 ) ;
#28260=VECTOR ( 'NONE', #14808, 39.37007874015748143 ) ;
#28317=EDGE_CURVE ( 'NONE', #19054, #28080, #30796, .T. ) ;
#28318=DIRECTION ( 'NONE',  ( -1.000000000000000000, 0.000000000000000000, 0.000000000000000000 ) ) ;
#28379=CARTESIAN_POINT ( 'NONE',  ( 0.000000000000000000, 0.4265678656643324129, 0.4783464566929144235 ) ) ;
#28408=AXIS2_PLACEMENT_3D ( 'NONE', #16045, #41870, #1634 ) ;
#28420=CARTESIAN_POINT ( 'NONE',  ( 0.000000000000000000, 0.4003652867858630282, 0.7276473417831955670 ) ) ;
#28447=ORIENTED_EDGE ( 'NONE', *, *, #12586, .T. ) ;
#28468=VERTEX_POINT ( 'NONE', #45590 ) ;
#28490=PLANE ( 'NONE',  #16875 ) ;
#28494=CIRCLE ( 'NONE', #11665, 0.02900000000000070230 ) ;
#28521=VECTOR ( 'NONE', #31947, 39.37007874015748143 ) ;
#28530=DIRECTION ( 'NONE',  ( -0.000000000000000000, 0.2126700594527843047, -0.9771240687918547607 ) ) ;
#28544=ADVANCED_FACE ( 'NONE', ( #23576 ), #44879, .T. ) ;
#28545=DIRECTION ( 'NONE',  ( 0.000000000000000000, -0.9771240687918547607, -0.2126700594527842492 ) ) ;
#28554=FACE_OUTER_BOUND ( 'NONE', #223, .T. ) ;
#28560=ORIENTED_EDGE ( 'NONE', *, *, #378, .T. ) ;
#28705=CARTESIAN_POINT ( 'NONE',  ( -0.1184675242425147629, -0.09842519685039370636, 2.185526306663016616 ) ) ;
#28719=PLANE ( 'NONE',  #38660 ) ;
#28720=ORIENTED_EDGE ( 'NONE', *, *, #25526, .T. ) ;
#28800=DIRECTION ( 'NONE',  ( 0.000000000000000000, 0.000000000000000000, 1.000000000000000000 ) ) ;
#28807=ORIENTED_EDGE ( 'NONE', *, *, #3268, .F. ) ;
#28808=AXIS2_PLACEMENT_3D ( 'NONE', #5972, #31646, #39263 ) ;
#28823=CYLINDRICAL_SURFACE ( 'NONE', #5752, 0.7874015748031437667 ) ;
#28858=ADVANCED_FACE ( 'NONE', ( #3877 ), #39813, .F. ) ;
#28892=ORIENTED_EDGE ( 'NONE', *, *, #24677, .T. ) ;
#28928=VERTEX_POINT ( 'NONE', #33385 ) ;
#28961=AXIS2_PLACEMENT_3D ( 'NONE', #22881, #16180, #12352 ) ;
#28975=CARTESIAN_POINT ( 'NONE',  ( -0.3161444924769509779, 2.177585298233989164, -3.731703755406937439 ) ) ;
#29028=AXIS2_PLACEMENT_3D ( 'NONE', #35858, #32290, #46162 ) ;
#29032=CARTESIAN_POINT ( 'NONE',  ( 0.03901279071809810040, -0.09842519685039370636, 1.224299699984025658 ) ) ;
#29047=ORIENTED_EDGE ( 'NONE', *, *, #10122, .T. ) ;
#29117=EDGE_CURVE ( 'NONE', #3012, #39709, #1216, .T. ) ;
#29162=DIRECTION ( 'NONE',  ( -3.532562060772668727E-15, 0.000000000000000000, 1.000000000000000000 ) ) ;
#29188=DIRECTION ( 'NONE',  ( -1.000000000000000000, 0.000000000000000000, 0.000000000000000000 ) ) ;
#29241=DIRECTION ( 'NONE',  ( -0.7986355100473023771, 5.219913244286809847E-16, -0.6018150231520357218 ) ) ;
#29299=ORIENTED_EDGE ( 'NONE', *, *, #17696, .F. ) ;
#29320=AXIS2_PLACEMENT_3D ( 'NONE', #1140, #1374, #34465 ) ;
#29370=CARTESIAN_POINT ( 'NONE',  ( 0.1574803149606299746, -5.122214988120488358E-16, -8.878505979408856939E-16 ) ) ;
#29384=ORIENTED_EDGE ( 'NONE', *, *, #1444, .T. ) ;
#29486=DIRECTION ( 'NONE',  ( 0.000000000000000000, 0.000000000000000000, -1.000000000000000000 ) ) ;
#29572=CARTESIAN_POINT ( 'NONE',  ( 0.1574803149606299746, -0.5708661417322835607, -6.991093932140394160E-17 ) ) ;
#29577=DIRECTION ( 'NONE',  ( -0.000000000000000000, -1.000000000000000000, -0.000000000000000000 ) ) ;
#29595=CARTESIAN_POINT ( 'NONE',  ( 0.1574803149606299746, -0.5708661417322837828, 2.134496832518260172E-17 ) ) ;
#29606=EDGE_CURVE ( 'NONE', #3438, #37269, #21088, .T. ) ;
#29631=PLANE ( 'NONE',  #34072 ) ;
#29661=DIRECTION ( 'NONE',  ( 0.000000000000000000, 0.000000000000000000, 1.000000000000000000 ) ) ;
#29665=ADVANCED_FACE ( 'NONE', ( #28554 ), #43123, .F. ) ;
#29678=ORIENTED_EDGE ( 'NONE', *, *, #31141, .F. ) ;
#29707=ORIENTED_EDGE ( 'NONE', *, *, #378, .F. ) ;
#29749=DIRECTION ( 'NONE',  ( 1.000000000000000000, 0.000000000000000000, 0.000000000000000000 ) ) ;
#29754=AXIS2_PLACEMENT_3D ( 'NONE', #5960, #5499, #16993 ) ;
#29757=EDGE_CURVE ( 'NONE', #26397, #35281, #9936, .T. ) ;
#29768=EDGE_CURVE ( 'NONE', #28928, #10268, #19880, .T. ) ;
#29784=AXIS2_PLACEMENT_3D ( 'NONE', #45027, #30942, #12727 ) ;
#29797=CARTESIAN_POINT ( 'NONE',  ( -0.1296641775163207277, 0.9382165298418964072, -1.070508272602716637 ) ) ;
#29855=FILL_AREA_STYLE ('',( #26706 ) ) ;
#29982=LINE ( 'NONE', #44998, #34504 ) ;
#29986=CARTESIAN_POINT ( 'NONE',  ( 0.1574803149606299746, 0.9876813667277571929, 0.7893767492247212303 ) ) ;
#30045=VERTEX_POINT ( 'NONE', #43548 ) ;
#30093=EDGE_CURVE ( 'NONE', #22445, #7415, #26044, .T. ) ;
#30096=( NAMED_UNIT ( * ) SI_UNIT ( $, .STERADIAN. ) SOLID_ANGLE_UNIT ( ) ) ;
#30158=DIRECTION ( 'NONE',  ( 0.000000000000000000, 0.000000000000000000, 1.000000000000000000 ) ) ;
#30161=CARTESIAN_POINT ( 'NONE',  ( -0.1586641775163213364, 1.025704337919491005, -1.138861239548321524 ) ) ;
#30181=ADVANCED_FACE ( 'NONE', ( #14572 ), #39949, .T. ) ;
#30198=ORIENTED_EDGE ( 'NONE', *, *, #14016, .T. ) ;
#30277=ORIENTED_EDGE ( 'NONE', *, *, #8336, .T. ) ;
#30278=AXIS2_PLACEMENT_3D ( 'NONE', #32293, #13577, #13818 ) ;
#30322=SURFACE_STYLE_FILL_AREA ( #29855 ) ;
#30485=DIRECTION ( 'NONE',  ( -0.000000000000000000, -0.2432573283306819767, 0.9699617890481142535 ) ) ;
#30522=VECTOR ( 'NONE', #21052, 39.37007874015748854 ) ;
#30527=DIRECTION ( 'NONE',  ( 1.000000000000000000, -0.000000000000000000, -0.000000000000000000 ) ) ;
#30577=ORIENTED_EDGE ( 'NONE', *, *, #40660, .T. ) ;
#30604=CARTESIAN_POINT ( 'NONE',  ( 0.04485236092672652969, 0.3740157480314960647, 1.206847064312616125 ) ) ;
#30626=VECTOR ( 'NONE', #22818, 39.37007874015748854 ) ;
#30674=CYLINDRICAL_SURFACE ( 'NONE', #28408, 0.3937007874015748254 ) ;
#30724=CARTESIAN_POINT ( 'NONE',  ( -0.1534195868007023067, 1.482597719745565312, -0.3467144894627436913 ) ) ;
#30732=LINE ( 'NONE', #12519, #23206 ) ;
#30756=VERTEX_POINT ( 'NONE', #42756 ) ;
#30785=CARTESIAN_POINT ( 'NONE',  ( 3.060083392313581123E-15, 0.5288907983920048128, -0.7507079620615672022 ) ) ;
#30796=LINE ( 'NONE', #26954, #6038 ) ;
#30814=DIRECTION ( 'NONE',  ( -1.000000000000000000, -0.000000000000000000, -0.000000000000000000 ) ) ;
#30847=DIRECTION ( 'NONE',  ( 0.000000000000000000, -1.000000000000000000, 0.000000000000000000 ) ) ;
#30882=DIRECTION ( 'NONE',  ( 0.000000000000000000, -0.7907053606985338101, 0.6121968903568536513 ) ) ;
#30942=DIRECTION ( 'NONE',  ( -1.000000000000000000, -0.000000000000000000, -0.000000000000000000 ) ) ;
#30945=CARTESIAN_POINT ( 'NONE',  ( -0.3161444924769509779, 1.209494567139720367, -1.479906699140297599 ) ) ;
#30986=VECTOR ( 'NONE', #21427, 39.37007874015748854 ) ;
#31002=SHAPE_DEFINITION_REPRESENTATION ( #21852, #43589 ) ;
#31022=ORIENTED_EDGE ( 'NONE', *, *, #31890, .F. ) ;
#31107=EDGE_LOOP ( 'NONE', ( #459, #41310, #6735, #21637, #28560, #5556, #30577, #28720, #2652, #14565, #39188 ) ) ;
#31114=PLANE ( 'NONE',  #35621 ) ;
#31133=ORIENTED_EDGE ( 'NONE', *, *, #47118, .F. ) ;
#31137=DIRECTION ( 'NONE',  ( 0.000000000000000000, 0.000000000000000000, -1.000000000000000000 ) ) ;
#31141=EDGE_CURVE ( 'NONE', #25222, #18796, #8110, .T. ) ;
#31142=LINE ( 'NONE', #35435, #22412 ) ;
#31157=ORIENTED_EDGE ( 'NONE', *, *, #41134, .F. ) ;
#31167=CARTESIAN_POINT ( 'NONE',  ( -0.1184675242425147629, -0.09842519685039369248, 1.555605046820496273 ) ) ;
#31183=CARTESIAN_POINT ( 'NONE',  ( -0.3161444924769509779, 1.205832402325951680, -1.129708666049261900 ) ) ;
#31202=ORIENTED_EDGE ( 'NONE', *, *, #45696, .F. ) ;
#31307=CARTESIAN_POINT ( 'NONE',  ( 0.06801279071811515420, -0.5708661417322834497, 1.224299699984019663 ) ) ;
#31344=CYLINDRICAL_SURFACE ( 'NONE', #4952, 0.3912448816427701037 ) ;
#31345=ADVANCED_FACE ( 'NONE', ( #10377 ), #2914, .T. ) ;
#31412=CYLINDRICAL_SURFACE ( 'NONE', #46304, 0.1574803149606292529 ) ;
#31413=DIMENSIONAL_EXPONENTS ( 1.000000000000000000, 0.000000000000000000, 0.000000000000000000, 0.000000000000000000, 0.000000000000000000, 0.000000000000000000, 0.000000000000000000 ) ;
#31505=CARTESIAN_POINT ( 'NONE',  ( 0.000000000000000000, -5.122214988120488358E-16, -8.878505979408856939E-16 ) ) ;
#31516=EDGE_CURVE ( 'NONE', #18913, #38550, #14440, .T. ) ;
#31547=CARTESIAN_POINT ( 'NONE',  ( -0.1184675242425147906, -0.09842519685039369248, 1.555605046820496273 ) ) ;
#31616=LINE ( 'NONE', #2345, #12363 ) ;
#31637=( GEOMETRIC_REPRESENTATION_CONTEXT ( 3 ) GLOBAL_UNCERTAINTY_ASSIGNED_CONTEXT ( ( #11990 ) ) GLOBAL_UNIT_ASSIGNED_CONTEXT ( ( #45107, #11611, #30096 ) ) REPRESENTATION_CONTEXT ( 'NONE', 'WORKASPACE' ) ) ;
#31646=DIRECTION ( 'NONE',  ( -1.000000000000000000, 0.000000000000000000, 0.000000000000000000 ) ) ;
#31662=DIRECTION ( 'NONE',  ( 0.6018150231520356108, -0.000000000000000000, -0.7986355100473022661 ) ) ;
#31676=ADVANCED_FACE ( 'NONE', ( #42108 ), #30674, .F. ) ;
#31700=ORIENTED_EDGE ( 'NONE', *, *, #8336, .F. ) ;
#31735=CIRCLE ( 'NONE', #37848, 0.02900000000000056352 ) ;
#31755=CARTESIAN_POINT ( 'NONE',  ( 1.530041696156790562E-15, 0.4667239666988196034, -0.7023826619074857724 ) ) ;
#31796=ADVANCED_FACE ( 'NONE', ( #20326 ), #34965, .F. ) ;
#31801=ORIENTED_EDGE ( 'NONE', *, *, #27123, .F. ) ;
#31862=EDGE_LOOP ( 'NONE', ( #28023, #8438, #5272, #36797, #40058, #42862, #17995, #13002, #2006, #41052 ) ) ;
#31890=EDGE_CURVE ( 'NONE', #8749, #7162, #13859, .T. ) ;
#31947=DIRECTION ( 'NONE',  ( 0.000000000000000000, 1.000000000000000000, 8.673617379884034486E-16 ) ) ;
#31965=VERTEX_POINT ( 'NONE', #18434 ) ;
#32054=DIRECTION ( 'NONE',  ( 1.000000000000000000, 0.000000000000000000, 0.000000000000000000 ) ) ;
#32063=ORIENTED_EDGE ( 'NONE', *, *, #39799, .T. ) ;
#32122=DIRECTION ( 'NONE',  ( -0.000000000000000000, 1.000000000000000000, 0.000000000000000000 ) ) ;
#32152=VECTOR ( 'NONE', #35940, 39.37007874015748143 ) ;
#32290=DIRECTION ( 'NONE',  ( 1.000000000000000000, 0.000000000000000000, 0.000000000000000000 ) ) ;
#32293=CARTESIAN_POINT ( 'NONE',  ( -0.1184675242425147629, -0.09842519685039370636, 1.713085361781126803 ) ) ;
#32298=AXIS2_PLACEMENT_3D ( 'NONE', #9308, #1868, #12452 ) ;
#32407=CIRCLE ( 'NONE', #3258, 0.02900000000000062597 ) ;
#32413=ORIENTED_EDGE ( 'NONE', *, *, #405, .F. ) ;
#32423=AXIS2_PLACEMENT_3D ( 'NONE', #31183, #4797, #19425 ) ;
#32487=DIRECTION ( 'NONE',  ( 1.000000000000000000, 0.000000000000000000, -0.000000000000000000 ) ) ;
#32497=DIRECTION ( 'NONE',  ( -0.000000000000000000, -1.000000000000000000, -0.000000000000000000 ) ) ;
#32593=ORIENTED_EDGE ( 'NONE', *, *, #26787, .F. ) ;
#32597=AXIS2_PLACEMENT_3D ( 'NONE', #6149, #1613, #17188 ) ;
#32612=DIRECTION ( 'NONE',  ( 0.000000000000000000, 1.000000000000000000, 0.000000000000000000 ) ) ;
#32649=VERTEX_POINT ( 'NONE', #23929 ) ;
#32652=DIRECTION ( 'NONE',  ( 0.000000000000000000, 0.000000000000000000, 1.000000000000000000 ) ) ;
#32778=AXIS2_PLACEMENT_3D ( 'NONE', #467, #8613, #33343 ) ;
#32803=DIRECTION ( 'NONE',  ( -0.000000000000000000, -1.000000000000000000, -0.000000000000000000 ) ) ;
#32848=PLANE ( 'NONE',  #35482 ) ;
#32851=ORIENTED_EDGE ( 'NONE', *, *, #29117, .F. ) ;
#32922=CIRCLE ( 'NONE', #711, 0.5708661417322833387 ) ;
#33013=AXIS2_PLACEMENT_3D ( 'NONE', #43351, #32612, #47199 ) ;
#33084=CARTESIAN_POINT ( 'NONE',  ( -0.1586641775163213364, 1.690605217543008632, -0.5092277576975117181 ) ) ;
#33089=ORIENTED_EDGE ( 'NONE', *, *, #29757, .F. ) ;
#33106=DIRECTION ( 'NONE',  ( 1.000000000000000000, 0.000000000000000000, 0.000000000000000000 ) ) ;
#33151=ORIENTED_EDGE ( 'NONE', *, *, #12809, .T. ) ;
#33184=ORIENTED_EDGE ( 'NONE', *, *, #29757, .T. ) ;
#33217=CARTESIAN_POINT ( 'NONE',  ( 0.1574803149606299746, 0.3883517482604934012, -0.6419475548153109612 ) ) ;
#33291=DIRECTION ( 'NONE',  ( 0.000000000000000000, -0.7880107536067225693, 0.6156614753256574035 ) ) ;
#33336=VERTEX_POINT ( 'NONE', #43650 ) ;
#33343=DIRECTION ( 'NONE',  ( 0.000000000000000000, 0.000000000000000000, -1.000000000000000000 ) ) ;
#33385=CARTESIAN_POINT ( 'NONE',  ( 0.1237557312196568837, 0.6131769916351970107, -0.8165595533554412810 ) ) ;
#33421=EDGE_CURVE ( 'NONE', #28468, #41308, #44509, .T. ) ;
#33447=CARTESIAN_POINT ( 'NONE',  ( 0.1574803149606299746, 1.086379535891617065, -0.03715491745705640919 ) ) ;
#33581=ADVANCED_FACE ( 'NONE', ( #27802 ), #12701, .T. ) ;
#33587=EDGE_LOOP ( 'NONE', ( #2751, #28892, #36800, #39141, #14870, #36344, #3230, #27930, #26154 ) ) ;
#33692=ORIENTED_EDGE ( 'NONE', *, *, #41363, .F. ) ;
#33705=ORIENTED_EDGE ( 'NONE', *, *, #36841, .F. ) ;
#33731=CARTESIAN_POINT ( 'NONE',  ( -0.02900000000000056352, 1.086379535891621506, -0.03715491745705966353 ) ) ;
#33751=EDGE_CURVE ( 'NONE', #10497, #34560, #47151, .T. ) ;
#33798=EDGE_CURVE ( 'NONE', #43609, #12706, #46661, .T. ) ;
#33807=ORIENTED_EDGE ( 'NONE', *, *, #19766, .F. ) ;
#33844=CARTESIAN_POINT ( 'NONE',  ( -0.1586641775163213364, 1.209494567139727250, -1.479906699140296045 ) ) ;
#33847=EDGE_CURVE ( 'NONE', #39709, #43013, #24632, .T. ) ;
#33870=VECTOR ( 'NONE', #21351, 39.37007874015748143 ) ;
#33937=VERTEX_POINT ( 'NONE', #30161 ) ;
#33946=CLOSED_SHELL ( 'NONE', ( #31676, #28858, #8696, #42014, #11186, #5189, #21657, #11267, #9819, #33581, #12495, #35225, #40075, #44563, #3896, #43504, #18393, #4425, #17264, #8489, #37226, #46361, #20072, #30181, #26093, #31345, #7768, #12705, #31796, #1025, #6263, #3950, #43337, #28544, #24310, #27954, #19860, #29665, #37992, #46747 ) ) ;
#33986=ORIENTED_EDGE ( 'NONE', *, *, #12809, .F. ) ;
#33987=CARTESIAN_POINT ( 'NONE',  ( 0.1574803149606299746, -0.5708661417322835607, 1.713085361781126803 ) ) ;
#33999=DIRECTION ( 'NONE',  ( 1.363218471095259303E-17, 0.6156614753256575145, 0.7880107536067225693 ) ) ;
#34016=FACE_OUTER_BOUND ( 'NONE', #19633, .T. ) ;
#34035=AXIS2_PLACEMENT_3D ( 'NONE', #38767, #35184, #43292 ) ;
#34057=CARTESIAN_POINT ( 'NONE',  ( -0.1586641775163213364, 1.798092712879851174, -3.826876940038414610 ) ) ;
#34061=CARTESIAN_POINT ( 'NONE',  ( 0.6656920301128459450, -0.5708661417322835607, 0.3829649962626329729 ) ) ;
#34072=AXIS2_PLACEMENT_3D ( 'NONE', #43705, #32487, #10669 ) ;
#34107=ORIENTED_EDGE ( 'NONE', *, *, #1994, .F. ) ;
#34125=CIRCLE ( 'NONE', #1972, 0.1864803149606299448 ) ;
#34129=CIRCLE ( 'NONE', #41703, 0.02900000000000052189 ) ;
#34150=LINE ( 'NONE', #20206, #20080 ) ;
#34175=CIRCLE ( 'NONE', #28808, 0.3937007874015748254 ) ;
#34251=CARTESIAN_POINT ( 'NONE',  ( 0.000000000000000000, 0.000000000000000000, 0.000000000000000000 ) ) ;
#34291=DIRECTION ( 'NONE',  ( -1.000000000000000000, -0.000000000000000000, -0.000000000000000000 ) ) ;
#34295=CARTESIAN_POINT ( 'NONE',  ( 0.03901279071809810040, 0.3740157480314960647, 1.713085361781127913 ) ) ;
#34444=ORIENTED_EDGE ( 'NONE', *, *, #29768, .T. ) ;
#34454=DIRECTION ( 'NONE',  ( 1.000000000000000000, -0.000000000000000000, -0.000000000000000000 ) ) ;
#34457=AXIS2_PLACEMENT_3D ( 'NONE', #43070, #29241, #25115 ) ;
#34458=EDGE_LOOP ( 'NONE', ( #46715, #19271, #39897, #33705 ) ) ;
#34465=DIRECTION ( 'NONE',  ( 0.000000000000000000, 0.000000000000000000, 1.000000000000000000 ) ) ;
#34504=VECTOR ( 'NONE', #1393, 39.37007874015748143 ) ;
#34559=DIRECTION ( 'NONE',  ( 0.6018150231520413840, -0.000000000000000000, -0.7986355100472980473 ) ) ;
#34560=VERTEX_POINT ( 'NONE', #10454 ) ;
#34566=ORIENTED_EDGE ( 'NONE', *, *, #14071, .T. ) ;
#34639=CARTESIAN_POINT ( 'NONE',  ( 0.1574803149606319730, 0.4667239666988196034, -0.7023826619074858835 ) ) ;
#34672=ORIENTED_EDGE ( 'NONE', *, *, #36848, .T. ) ;
#34697=LINE ( 'NONE', #41836, #3839 ) ;
#34704=VECTOR ( 'NONE', #31662, 39.37007874015748854 ) ;
#34750=ORIENTED_EDGE ( 'NONE', *, *, #15820, .F. ) ;
#34812=ORIENTED_EDGE ( 'NONE', *, *, #24843, .F. ) ;
#34894=CARTESIAN_POINT ( 'NONE',  ( -0.1184675242425147906, -0.09842519685039370636, 1.870565676741754668 ) ) ;
#34939=DIRECTION ( 'NONE',  ( 0.000000000000000000, 0.000000000000000000, -1.000000000000000000 ) ) ;
#34965=CYLINDRICAL_SURFACE ( 'NONE', #21476, 0.2952755905511806334 ) ;
#34996=CYLINDRICAL_SURFACE ( 'NONE', #29784, 0.1574803149606292529 ) ;
#35048=ORIENTED_EDGE ( 'NONE', *, *, #16236, .T. ) ;
#35075=DIRECTION ( 'NONE',  ( -0.000000000000000000, 0.7880107536067174623, -0.6156614753256640649 ) ) ;
#35114=ORIENTED_EDGE ( 'NONE', *, *, #6147, .F. ) ;
#35127=CARTESIAN_POINT ( 'NONE',  ( -0.3161444924769509779, 2.559880088878760951, -3.648497683167374550 ) ) ;
#35171=ORIENTED_EDGE ( 'NONE', *, *, #25617, .T. ) ;
#35184=DIRECTION ( 'NONE',  ( 1.000000000000000000, 0.000000000000000000, 0.000000000000000000 ) ) ;
#35225=ADVANCED_FACE ( 'NONE', ( #14696 ), #518, .T. ) ;
#35239=VECTOR ( 'NONE', #34291, 39.37007874015748143 ) ;
#35281=VERTEX_POINT ( 'NONE', #19449 ) ;
#35312=DIRECTION ( 'NONE',  ( 0.6018150231520412730, 0.000000000000000000, -0.7986355100472980473 ) ) ;
#35420=DIRECTION ( 'NONE',  ( 0.000000000000000000, -0.7907053606985338101, 0.6121968903568536513 ) ) ;
#35431=DIRECTION ( 'NONE',  ( 0.000000000000000000, 0.6156614753256575145, 0.7880107536067224583 ) ) ;
#35435=CARTESIAN_POINT ( 'NONE',  ( -0.3161444924769541420, 0.8918838478058933594, -1.034309214090480822 ) ) ;
#35482=AXIS2_PLACEMENT_3D ( 'NONE', #11030, #28545, #10560 ) ;
#35517=ORIENTED_EDGE ( 'NONE', *, *, #16236, .F. ) ;
#35561=CIRCLE ( 'NONE', #27943, 0.3912448816427701037 ) ;
#35621=AXIS2_PLACEMENT_3D ( 'NONE', #45679, #23435, #5442 ) ;
#35675=DIRECTION ( 'NONE',  ( 0.000000000000000000, 1.000000000000000000, 0.000000000000000000 ) ) ;
#35690=EDGE_CURVE ( 'NONE', #36971, #44905, #9066, .T. ) ;
#35719=EDGE_CURVE ( 'NONE', #40831, #45750, #8347, .T. ) ;
#35749=ORIENTED_EDGE ( 'NONE', *, *, #2644, .F. ) ;
#35751=CARTESIAN_POINT ( 'NONE',  ( 0.1574803149606299746, -0.09842519685039370636, 2.185526306663016616 ) ) ;
#35765=AXIS2_PLACEMENT_3D ( 'NONE', #44657, #30814, #18804 ) ;
#35858=CARTESIAN_POINT ( 'NONE',  ( 0.03901279071809810040, -0.09842519685039370636, 1.713085361781125471 ) ) ;
#35905=ORIENTED_EDGE ( 'NONE', *, *, #13144, .T. ) ;
#35923=EDGE_LOOP ( 'NONE', ( #18530, #46281, #38702, #24602, #35517, #11783, #8370, #18402, #11468, #42630, #31202, #22065 ) ) ;
#35940=DIRECTION ( 'NONE',  ( -0.000000000000000000, -1.000000000000000000, -8.673617379884034486E-16 ) ) ;
#36032=MANIFOLD_SOLID_BREP ( 'Handle Arm Left', #33946 ) ;
#36037=AXIS2_PLACEMENT_3D ( 'NONE', #15169, #40760, #22807 ) ;
#36071=DIRECTION ( 'NONE',  ( 0.000000000000000000, -0.7880107536067204599, 0.6156614753256602901 ) ) ;
#36101=CARTESIAN_POINT ( 'NONE',  ( 0.1099139000111727243, -0.5708661417322835607, 1.120507485783946100 ) ) ;
#36136=DIRECTION ( 'NONE',  ( 0.000000000000000000, 0.000000000000000000, 1.000000000000000000 ) ) ;
#36139=CIRCLE ( 'NONE', #13963, 0.02900000000000064679 ) ;
#36190=ORIENTED_EDGE ( 'NONE', *, *, #28317, .T. ) ;
#36232=DIRECTION ( 'NONE',  ( 0.000000000000000000, 0.000000000000000000, -1.000000000000000000 ) ) ;
#36344=ORIENTED_EDGE ( 'NONE', *, *, #10580, .T. ) ;
#36362=ORIENTED_EDGE ( 'NONE', *, *, #13121, .F. ) ;
#36382=EDGE_CURVE ( 'NONE', #41308, #22445, #9894, .T. ) ;
#36459=EDGE_LOOP ( 'NONE', ( #11407, #2090, #3503, #30198 ) ) ;
#36489=CARTESIAN_POINT ( 'NONE',  ( 0.04485236092672649499, -0.5708661417322835607, 1.206847064312616125 ) ) ;
#36647=AXIS2_PLACEMENT_3D ( 'NONE', #13384, #42799, #31137 ) ;
#36655=FACE_OUTER_BOUND ( 'NONE', #42503, .T. ) ;
#36680=CARTESIAN_POINT ( 'NONE',  ( -0.3161444924769509779, 1.690605217543007077, -0.5092277576975137166 ) ) ;
#36691=VECTOR ( 'NONE', #20236, 39.37007874015748854 ) ;
#36701=FACE_OUTER_BOUND ( 'NONE', #47198, .T. ) ;
#36707=AXIS2_PLACEMENT_3D ( 'NONE', #15829, #41406, #5011 ) ;
#36724=ORIENTED_EDGE ( 'NONE', *, *, #19643, .F. ) ;
#36780=AXIS2_PLACEMENT_3D ( 'NONE', #45825, #21137, #35312 ) ;
#36797=ORIENTED_EDGE ( 'NONE', *, *, #30093, .T. ) ;
#36800=ORIENTED_EDGE ( 'NONE', *, *, #4750, .T. ) ;
#36841=EDGE_CURVE ( 'NONE', #3105, #43609, #10803, .T. ) ;
#36848=EDGE_CURVE ( 'NONE', #12706, #14162, #895, .T. ) ;
#36870=EDGE_LOOP ( 'NONE', ( #25662, #17359, #5512, #46427 ) ) ;
#36879=CARTESIAN_POINT ( 'NONE',  ( 0.000000000000000000, 0.08719492171395763769, -0.5641677032617172793 ) ) ;
#36916=EDGE_CURVE ( 'NONE', #17177, #4491, #14910, .T. ) ;
#36949=DIRECTION ( 'NONE',  ( 0.000000000000000000, 0.000000000000000000, -1.000000000000000000 ) ) ;
#36960=AXIS2_PLACEMENT_3D ( 'NONE', #46189, #35431, #6876 ) ;
#36971=VERTEX_POINT ( 'NONE', #37171 ) ;
#36995=VERTEX_POINT ( 'NONE', #30724 ) ;
#36998=FACE_BOUND ( 'NONE', #8096, .T. ) ;
#37042=ORIENTED_EDGE ( 'NONE', *, *, #35690, .F. ) ;
#37047=CARTESIAN_POINT ( 'NONE',  ( -0.005244590715619158044, 1.099487083487566297, -0.04739565599251693157 ) ) ;
#37106=EDGE_CURVE ( 'NONE', #34560, #7415, #2163, .T. ) ;
#37171=CARTESIAN_POINT ( 'NONE',  ( -0.3161444924769509779, 2.177585298233989164, -4.122948637049707266 ) ) ;
#37226=ADVANCED_FACE ( 'NONE', ( #36655 ), #32848, .F. ) ;
#37229=SURFACE_STYLE_USAGE ( .BOTH. , #15204 ) ;
#37252=FACE_BOUND ( 'NONE', #37931, .T. ) ;
#37269=VERTEX_POINT ( 'NONE', #33084 ) ;
#37385=ORIENTED_EDGE ( 'NONE', *, *, #41363, .T. ) ;
#37417=CIRCLE ( 'NONE', #8343, 0.5708661417322833387 ) ;
#37455=VECTOR ( 'NONE', #25426, 39.37007874015748143 ) ;
#37518=DIRECTION ( 'NONE',  ( -2.775557561562890735E-17, 0.6156614753256639538, 0.7880107536067174623 ) ) ;
#37533=CARTESIAN_POINT ( 'NONE',  ( -0.3161444924769509779, 0.4457451269443606368, -1.671447902550282194 ) ) ;
#37583=ORIENTED_EDGE ( 'NONE', *, *, #13909, .T. ) ;
#37595=VECTOR ( 'NONE', #1316, 39.37007874015748143 ) ;
#37670=VECTOR ( 'NONE', #13272, 39.37007874015748143 ) ;
#37718=EDGE_LOOP ( 'NONE', ( #34750, #3911, #24363, #26486 ) ) ;
#37753=CARTESIAN_POINT ( 'NONE',  ( 0.1574803149606299746, 0.1473293504822046074, -0.5595480905233950475 ) ) ;
#37781=DIRECTION ( 'NONE',  ( 1.000000000000000000, -0.000000000000000000, -0.000000000000000000 ) ) ;
#37848=AXIS2_PLACEMENT_3D ( 'NONE', #46708, #39520, #21312 ) ;
#37931=EDGE_LOOP ( 'NONE', ( #17894, #5457 ) ) ;
#37963=CARTESIAN_POINT ( 'NONE',  ( 0.000000000000000000, -0.5708661417322837828, 2.134496832518260172E-17 ) ) ;
#37992=ADVANCED_FACE ( 'NONE', ( #679 ), #11983, .F. ) ;
#38023=LINE ( 'NONE', #27751, #422 ) ;
#38042=DIRECTION ( 'NONE',  ( 0.5735764363510331698, -0.6455006197386610189, 0.5043203561029969695 ) ) ;
#38131=DIRECTION ( 'NONE',  ( 0.5735764363510332808, -0.6455006197386610189, 0.5043203561029969695 ) ) ;
#38146=ORIENTED_EDGE ( 'NONE', *, *, #15233, .F. ) ;
#38195=AXIS2_PLACEMENT_3D ( 'NONE', #8539, #9018, #23172 ) ;
#38275=CARTESIAN_POINT ( 'NONE',  ( -0.3161444924769509779, 1.449372585305505723, -0.3207561694859716317 ) ) ;
#38435=ORIENTED_EDGE ( 'NONE', *, *, #9114, .F. ) ;
#38469=EDGE_CURVE ( 'NONE', #34560, #11282, #34125, .T. ) ;
#38550=VERTEX_POINT ( 'NONE', #8071 ) ;
#38660=AXIS2_PLACEMENT_3D ( 'NONE', #42565, #13830, #38765 ) ;
#38661=LINE ( 'NONE', #45587, #22233 ) ;
#38702=ORIENTED_EDGE ( 'NONE', *, *, #12586, .F. ) ;
#38719=PLANE ( 'NONE',  #25948 ) ;
#38722=DIRECTION ( 'NONE',  ( 0.000000000000000000, 1.000000000000000000, 8.673617379884034486E-16 ) ) ;
#38765=DIRECTION ( 'NONE',  ( 0.000000000000000000, -0.000000000000000000, 1.000000000000000000 ) ) ;
#38767=CARTESIAN_POINT ( 'NONE',  ( 0.03901279071809810040, -0.09842519685039370636, 1.713085361781127913 ) ) ;
#38776=CARTESIAN_POINT ( 'NONE',  ( 3.060083392313581123E-15, 0.9310112235910578127, -1.064878870394357468 ) ) ;
#38804=EDGE_CURVE ( 'NONE', #23245, #30756, #38023, .T. ) ;
#38816=ORIENTED_EDGE ( 'NONE', *, *, #36848, .F. ) ;
#38916=DIRECTION ( 'NONE',  ( -5.934354299241488461E-32, -1.000000000000000000, -8.673617379884034486E-16 ) ) ;
#38967=VECTOR ( 'NONE', #38916, 39.37007874015748143 ) ;
#39005=DIRECTION ( 'NONE',  ( -1.000000000000000000, 0.000000000000000000, 0.000000000000000000 ) ) ;
#39037=ORIENTED_EDGE ( 'NONE', *, *, #23709, .T. ) ;
#39040=LINE ( 'NONE', #17475, #6436 ) ;
#39050=VECTOR ( 'NONE', #7874, 39.37007874015748143 ) ;
#39141=ORIENTED_EDGE ( 'NONE', *, *, #41134, .T. ) ;
#39155=AXIS2_PLACEMENT_3D ( 'NONE', #42366, #39005, #20794 ) ;
#39169=CARTESIAN_POINT ( 'NONE',  ( 0.06801279071811515420, -0.09842519685039327615, 1.224299699984020107 ) ) ;
#39188=ORIENTED_EDGE ( 'NONE', *, *, #40888, .T. ) ;
#39203=ORIENTED_EDGE ( 'NONE', *, *, #29606, .F. ) ;
#39214=DIRECTION ( 'NONE',  ( 0.000000000000000000, 1.000000000000000000, 8.673617379884034486E-16 ) ) ;
#39217=ORIENTED_EDGE ( 'NONE', *, *, #29768, .F. ) ;
#39260=LINE ( 'NONE', #6671, #30522 ) ;
#39263=DIRECTION ( 'NONE',  ( 0.000000000000000000, 0.000000000000000000, 1.000000000000000000 ) ) ;
#39284=DIRECTION ( 'NONE',  ( 1.000000000000000000, -0.000000000000000000, -0.000000000000000000 ) ) ;
#39311=EDGE_LOOP ( 'NONE', ( #11172, #12131, #10602, #32851 ) ) ;
#39413=VERTEX_POINT ( 'NONE', #12022 ) ;
#39470=DIRECTION ( 'NONE',  ( 1.000000000000000000, -0.000000000000000000, -0.000000000000000000 ) ) ;
#39516=VERTEX_POINT ( 'NONE', #22795 ) ;
#39520=DIRECTION ( 'NONE',  ( -0.000000000000000000, 1.000000000000000000, -0.000000000000000000 ) ) ;
#39534=DIRECTION ( 'NONE',  ( -1.000000000000000000, 0.000000000000000000, 0.000000000000000000 ) ) ;
#39626=FACE_OUTER_BOUND ( 'NONE', #41765, .T. ) ;
#39689=CYLINDRICAL_SURFACE ( 'NONE', #36960, 0.02900000000000054270 ) ;
#39709=VERTEX_POINT ( 'NONE', #40042 ) ;
#39726=VECTOR ( 'NONE', #41205, 39.37007874015748143 ) ;
#39780=CARTESIAN_POINT ( 'NONE',  ( -0.3161444924769509779, 0.4457451269443606368, -1.671447902550282194 ) ) ;
#39799=EDGE_CURVE ( 'NONE', #4833, #44905, #40447, .T. ) ;
#39813=CYLINDRICAL_SURFACE ( 'NONE', #19835, 0.2952755905511806334 ) ;
#39887=ORIENTED_EDGE ( 'NONE', *, *, #22296, .T. ) ;
#39897=ORIENTED_EDGE ( 'NONE', *, *, #21866, .F. ) ;
#39912=CARTESIAN_POINT ( 'NONE',  ( -0.1586641775163213364, 2.177585298233989164, -4.122948637049707266 ) ) ;
#39943=VECTOR ( 'NONE', #20883, 39.37007874015748143 ) ;
#39949=PLANE ( 'NONE',  #34457 ) ;
#39972=VERTEX_POINT ( 'NONE', #6166 ) ;
#39986=LINE ( 'NONE', #3810, #19229 ) ;
#40007=ORIENTED_EDGE ( 'NONE', *, *, #24677, .F. ) ;
#40022=CARTESIAN_POINT ( 'NONE',  ( -0.2824199087359778870, 1.411419074098322346, -0.2911036367043326467 ) ) ;
#40042=CARTESIAN_POINT ( 'NONE',  ( 0.000000000000000000, 0.3883517482604934012, -0.6419475548153109612 ) ) ;
#40058=ORIENTED_EDGE ( 'NONE', *, *, #37106, .F. ) ;
#40075=ADVANCED_FACE ( 'NONE', ( #24566 ), #38719, .T. ) ;
#40086=VERTEX_POINT ( 'NONE', #31547 ) ;
#40153=ORIENTED_EDGE ( 'NONE', *, *, #28317, .F. ) ;
#40193=CARTESIAN_POINT ( 'NONE',  ( 0.03901279071809810040, -0.5708661417322835607, 1.713085361781127913 ) ) ;
#40200=LINE ( 'NONE', #14362, #23446 ) ;
#40415=LINE ( 'NONE', #33987, #15286 ) ;
#40447=CIRCLE ( 'NONE', #36647, 0.3912448816427701037 ) ;
#40538=EDGE_CURVE ( 'NONE', #13132, #46787, #22030, .T. ) ;
#40542=ORIENTED_EDGE ( 'NONE', *, *, #47057, .F. ) ;
#40550=EDGE_CURVE ( 'NONE', #16648, #44831, #44961, .T. ) ;
#40566=CARTESIAN_POINT ( 'NONE',  ( 0.1237557312196567866, 0.6131769916351965666, -0.8165595533554419472 ) ) ;
#40620=DIRECTION ( 'NONE',  ( 0.000000000000000000, 0.000000000000000000, -1.000000000000000000 ) ) ;
#40660=EDGE_CURVE ( 'NONE', #26397, #24855, #12573, .T. ) ;
#40691=ORIENTED_EDGE ( 'NONE', *, *, #25617, .F. ) ;
#40760=DIRECTION ( 'NONE',  ( 0.000000000000000000, 0.9699617890481143645, 0.2432573283306820044 ) ) ;
#40831=VERTEX_POINT ( 'NONE', #1507 ) ;
#40867=ORIENTED_EDGE ( 'NONE', *, *, #25526, .F. ) ;
#40888=EDGE_CURVE ( 'NONE', #25222, #22261, #37417, .T. ) ;
#40891=FACE_OUTER_BOUND ( 'NONE', #17354, .T. ) ;
#40908=AXIS2_PLACEMENT_3D ( 'NONE', #23249, #33106, #14876 ) ;
#40923=ORIENTED_EDGE ( 'NONE', *, *, #23709, .F. ) ;
#40959=CARTESIAN_POINT ( 'NONE',  ( 0.000000000000000000, 0.1473293504822046074, -0.5595480905233950475 ) ) ;
#40967=DIRECTION ( 'NONE',  ( 1.000000000000000000, -0.000000000000000000, -0.000000000000000000 ) ) ;
#41004=ORIENTED_EDGE ( 'NONE', *, *, #11885, .F. ) ;
#41052=ORIENTED_EDGE ( 'NONE', *, *, #21866, .T. ) ;
#41131=ORIENTED_EDGE ( 'NONE', *, *, #10512, .F. ) ;
#41134=EDGE_CURVE ( 'NONE', #41392, #36971, #35561, .T. ) ;
#41152=VECTOR ( 'NONE', #21261, 39.37007874015748143 ) ;
#41205=DIRECTION ( 'NONE',  ( -1.000000000000000000, -0.000000000000000000, -0.000000000000000000 ) ) ;
#41236=PLANE ( 'NONE',  #42615 ) ;
#41308=VERTEX_POINT ( 'NONE', #15979 ) ;
#41310=ORIENTED_EDGE ( 'NONE', *, *, #36382, .T. ) ;
#41320=DIRECTION ( 'NONE',  ( -1.000000000000000000, 0.000000000000000000, 0.000000000000000000 ) ) ;
#41363=EDGE_CURVE ( 'NONE', #46267, #33937, #14897, .T. ) ;
#41392=VERTEX_POINT ( 'NONE', #35127 ) ;
#41406=DIRECTION ( 'NONE',  ( 1.217491584052838080E-15, 0.6156614753256588468, 0.7880107536067214591 ) ) ;
#41413=FACE_BOUND ( 'NONE', #27537, .T. ) ;
#41459=VECTOR ( 'NONE', #5160, 39.37007874015748143 ) ;
#41487=AXIS2_PLACEMENT_3D ( 'NONE', #558, #15214, #44407 ) ;
#41491=CARTESIAN_POINT ( 'NONE',  ( 0.03901279071809810040, 0.3740157480314960647, 1.224299699984025658 ) ) ;
#41537=AXIS2_PLACEMENT_3D ( 'NONE', #46699, #46229, #10548 ) ;
#41633=AXIS2_PLACEMENT_3D ( 'NONE', #45578, #39284, #21076 ) ;
#41639=CARTESIAN_POINT ( 'NONE',  ( 0.1099139000111727937, -0.5708661417322835607, 1.120507485783946100 ) ) ;
#41703=AXIS2_PLACEMENT_3D ( 'NONE', #10715, #6847, #21465 ) ;
#41752=CARTESIAN_POINT ( 'NONE',  ( -0.1296641775163210608, 0.1169123912647635627, -2.121729632260043186 ) ) ;
#41765=EDGE_LOOP ( 'NONE', ( #12662, #44412, #15923, #6823, #25429 ) ) ;
#41807=DIRECTION ( 'NONE',  ( 0.000000000000000000, -0.6121968903568536513, -0.7907053606985338101 ) ) ;
#41828=VERTEX_POINT ( 'NONE', #248 ) ;
#41836=CARTESIAN_POINT ( 'NONE',  ( 0.1574803149606299746, -0.5708661417322837828, 2.134496832518260172E-17 ) ) ;
#41838=LINE ( 'NONE', #15786, #42731 ) ;
#41870=DIRECTION ( 'NONE',  ( -1.000000000000000000, 0.000000000000000000, 0.000000000000000000 ) ) ;
#41971=AXIS2_PLACEMENT_3D ( 'NONE', #41752, #23348, #8956 ) ;
#42014=ADVANCED_FACE ( 'NONE', ( #16714 ), #31344, .T. ) ;
#42108=FACE_OUTER_BOUND ( 'NONE', #39311, .T. ) ;
#42238=DIRECTION ( 'NONE',  ( -0.000000000000000000, -0.7880107536067214591, 0.6156614753256588468 ) ) ;
#42269=VERTEX_POINT ( 'NONE', #20763 ) ;
#42358=PLANE ( 'NONE',  #24712 ) ;
#42366=CARTESIAN_POINT ( 'NONE',  ( 0.1574803149606299746, -0.09842519685039370636, 1.713085361781126803 ) ) ;
#42503=EDGE_LOOP ( 'NONE', ( #13619, #18233, #26319, #5954 ) ) ;
#42544=EDGE_LOOP ( 'NONE', ( #33089, #38435, #40542, #10957 ) ) ;
#42565=CARTESIAN_POINT ( 'NONE',  ( 0.1574803149606299746, 0.3740157480314960647, 1.713085361781126803 ) ) ;
#42584=CARTESIAN_POINT ( 'NONE',  ( -0.3161444924769509779, 1.798092712879851174, -3.826876940038414610 ) ) ;
#42615=AXIS2_PLACEMENT_3D ( 'NONE', #23073, #11501, #22036 ) ;
#42630=ORIENTED_EDGE ( 'NONE', *, *, #33421, .T. ) ;
#42653=ORIENTED_EDGE ( 'NONE', *, *, #31516, .T. ) ;
#42662=ORIENTED_EDGE ( 'NONE', *, *, #17696, .T. ) ;
#42731=VECTOR ( 'NONE', #33999, 39.37007874015748854 ) ;
#42756=CARTESIAN_POINT ( 'NONE',  ( 0.1574803149606300023, 0.000000000000000000, -0.2952755905511806334 ) ) ;
#42786=PLANE ( 'NONE',  #427 ) ;
#42799=DIRECTION ( 'NONE',  ( -1.000000000000000000, 0.000000000000000000, 0.000000000000000000 ) ) ;
#42846=APPLICATION_CONTEXT ( 'automotive_design' ) ;
#42862=ORIENTED_EDGE ( 'NONE', *, *, #38469, .T. ) ;
#42886=ORIENTED_EDGE ( 'NONE', *, *, #1494, .F. ) ;
#42926=CARTESIAN_POINT ( 'NONE',  ( -0.3161444924769509779, 1.209494567139720367, -1.479906699140297599 ) ) ;
#42951=DIRECTION ( 'NONE',  ( -1.000000000000000000, 0.000000000000000000, 0.000000000000000000 ) ) ;
#42977=EDGE_CURVE ( 'NONE', #28080, #9213, #4990, .T. ) ;
#43013=VERTEX_POINT ( 'NONE', #40959 ) ;
#43059=CARTESIAN_POINT ( 'NONE',  ( 0.000000000000000000, 0.1473293504822046074, -0.9532488779249699284 ) ) ;
#43061=CARTESIAN_POINT ( 'NONE',  ( -0.1586641775163213364, 2.177585298233989164, -3.731703755406937439 ) ) ;
#43070=CARTESIAN_POINT ( 'NONE',  ( -0.1184675242425147629, -0.5708661417322835607, 1.161904259418922170 ) ) ;
#43123=CYLINDRICAL_SURFACE ( 'NONE', #696, 0.3937007874015748254 ) ;
#43130=DIRECTION ( 'NONE',  ( -1.000000000000000000, 0.000000000000000000, 0.000000000000000000 ) ) ;
#43167=DIRECTION ( 'NONE',  ( 0.000000000000000000, 0.000000000000000000, 1.000000000000000000 ) ) ;
#43207=EDGE_CURVE ( 'NONE', #31965, #30756, #43265, .T. ) ;
#43265=CIRCLE ( 'NONE', #32597, 0.2952755905511806334 ) ;
#43288=CARTESIAN_POINT ( 'NONE',  ( 0.03901279071809810040, -0.09842519685039370636, 1.713085361781125471 ) ) ;
#43292=DIRECTION ( 'NONE',  ( 0.000000000000000000, 0.000000000000000000, -1.000000000000000000 ) ) ;
#43308=CARTESIAN_POINT ( 'NONE',  ( 0.06801279071811515420, 0.3740157480314961203, 1.224299699984020551 ) ) ;
#43313=DIRECTION ( 'NONE',  ( -8.890457814381144247E-15, 0.000000000000000000, 1.000000000000000000 ) ) ;
#43337=ADVANCED_FACE ( 'NONE', ( #3269 ), #10487, .F. ) ;
#43351=CARTESIAN_POINT ( 'NONE',  ( -0.07874015748031489015, 0.3740157480314960647, 0.9783464566929127582 ) ) ;
#43413=DIRECTION ( 'NONE',  ( -1.000000000000000000, 0.000000000000000000, 0.000000000000000000 ) ) ;
#43493=EDGE_CURVE ( 'NONE', #40831, #32649, #44820, .T. ) ;
#43504=ADVANCED_FACE ( 'NONE', ( #17895 ), #42786, .T. ) ;
#43534=FACE_BOUND ( 'NONE', #9526, .T. ) ;
#43539=AXIS2_PLACEMENT_3D ( 'NONE', #26476, #26715, #8235 ) ;
#43548=CARTESIAN_POINT ( 'NONE',  ( -0.1586641775163213364, 0.9382165298418959631, -1.070508272602717303 ) ) ;
#43580=AXIS2_PLACEMENT_3D ( 'NONE', #3726, #29188, #29661 ) ;
#43589=SHAPE_REPRESENTATION ( 'Handle Arm Left', ( #20860 ), #187 ) ;
#43592=DIRECTION ( 'NONE',  ( 0.000000000000000000, 0.000000000000000000, -1.000000000000000000 ) ) ;
#43609=VERTEX_POINT ( 'NONE', #41491 ) ;
#43650=CARTESIAN_POINT ( 'NONE',  ( 0.1574803149606299746, 0.3740157480314960647, 0.9783464566929134243 ) ) ;
#43705=CARTESIAN_POINT ( 'NONE',  ( -0.1184675242425147629, -0.09842519685039370636, 1.713085361781126803 ) ) ;
#43775=LINE ( 'NONE', #10978, #23905 ) ;
#43796=ORIENTED_EDGE ( 'NONE', *, *, #29117, .T. ) ;
#43814=CIRCLE ( 'NONE', #41487, 0.7874015748031497619 ) ;
#43857=VECTOR ( 'NONE', #13288, 39.37007874015748854 ) ;
#43863=FACE_OUTER_BOUND ( 'NONE', #35923, .T. ) ;
#43876=( LENGTH_UNIT ( ) NAMED_UNIT ( * ) SI_UNIT ( $, .METRE. ) ) ;
#43961=CIRCLE ( 'NONE', #23317, 0.1574803149606292529 ) ;
#44016=DIRECTION ( 'NONE',  ( 0.000000000000000000, 0.000000000000000000, 1.000000000000000000 ) ) ;
#44062=DIRECTION ( 'NONE',  ( -0.000000000000000000, 0.2126700594527843047, -0.9771240687918547607 ) ) ;
#44084=EDGE_CURVE ( 'NONE', #6378, #3012, #34175, .T. ) ;
#44136=EDGE_LOOP ( 'NONE', ( #35905, #43796, #40867, #4305 ) ) ;
#44270=ORIENTED_EDGE ( 'NONE', *, *, #10580, .F. ) ;
#44286=VECTOR ( 'NONE', #30882, 39.37007874015748143 ) ;
#44328=AXIS2_PLACEMENT_3D ( 'NONE', #10651, #3676, #14952 ) ;
#44329=EDGE_CURVE ( 'NONE', #10268, #47403, #40200, .T. ) ;
#44335=CARTESIAN_POINT ( 'NONE',  ( 0.1574803149606299746, -0.5708661417322835607, 0.9783464566929124251 ) ) ;
#44407=DIRECTION ( 'NONE',  ( 0.000000000000000000, 0.000000000000000000, -1.000000000000000000 ) ) ;
#44412=ORIENTED_EDGE ( 'NONE', *, *, #2320, .T. ) ;
#44488=LINE ( 'NONE', #40193, #4566 ) ;
#44505=EDGE_CURVE ( 'NONE', #39972, #23980, #8563, .T. ) ;
#44509=CIRCLE ( 'NONE', #7009, 0.07874015748031489015 ) ;
#44563=ADVANCED_FACE ( 'NONE', ( #9046 ), #31114, .T. ) ;
#44564=ORIENTED_EDGE ( 'NONE', *, *, #3692, .T. ) ;
#44617=CIRCLE ( 'NONE', #32423, 0.7874015748031497619 ) ;
#44657=CARTESIAN_POINT ( 'NONE',  ( -0.1184675242425147906, -0.09842519685039370636, 1.713085361781125471 ) ) ;
#44685=DIRECTION ( 'NONE',  ( 7.065124121545350864E-15, -0.7880107536067211260, 0.6156614753256594019 ) ) ;
#44764=FACE_OUTER_BOUND ( 'NONE', #19762, .T. ) ;
#44807=EDGE_CURVE ( 'NONE', #44831, #39516, #24136, .T. ) ;
#44820=CIRCLE ( 'NONE', #24944, 0.1574803149606292529 ) ;
#44821=ORIENTED_EDGE ( 'NONE', *, *, #38804, .F. ) ;
#44831=VERTEX_POINT ( 'NONE', #28705 ) ;
#44879=CYLINDRICAL_SURFACE ( 'NONE', #41971, 0.1864803149606298338 ) ;
#44902=LINE ( 'NONE', #12598, #12071 ) ;
#44905=VERTEX_POINT ( 'NONE', #39912 ) ;
#44910=VECTOR ( 'NONE', #30527, 39.37007874015748143 ) ;
#44935=CIRCLE ( 'NONE', #35765, 0.1574803149606292529 ) ;
#44961=CIRCLE ( 'NONE', #12855, 0.4724409448818896462 ) ;
#44989=EDGE_LOOP ( 'NONE', ( #923, #2465, #19139, #23186 ) ) ;
#44998=CARTESIAN_POINT ( 'NONE',  ( 0.1574803149606299746, -5.122214988120488358E-16, 0.9783464566929127582 ) ) ;
#45027=CARTESIAN_POINT ( 'NONE',  ( -0.1184675242425147629, -0.09842519685039370636, 1.713085361781125471 ) ) ;
#45057=LINE ( 'NONE', #12037, #9422 ) ;
#45107=( CONVERSION_BASED_UNIT ( 'INCH', #1029 ) LENGTH_UNIT ( ) NAMED_UNIT ( #31413 ) ) ;
#45135=CYLINDRICAL_SURFACE ( 'NONE', #28961, 0.4724409448818896462 ) ;
#45141=ORIENTED_EDGE ( 'NONE', *, *, #16377, .T. ) ;
#45232=CARTESIAN_POINT ( 'NONE',  ( 0.1574803149606299746, 0.4265678656643324129, 0.4783464566929144235 ) ) ;
#45246=DIRECTION ( 'NONE',  ( 0.000000000000000000, 1.000000000000000000, 0.000000000000000000 ) ) ;
#45319=LINE ( 'NONE', #9151, #5330 ) ;
#45326=ORIENTED_EDGE ( 'NONE', *, *, #26152, .F. ) ;
#45332=LINE ( 'NONE', #20173, #44910 ) ;
#45374=ORIENTED_EDGE ( 'NONE', *, *, #13144, .F. ) ;
#45450=ORIENTED_EDGE ( 'NONE', *, *, #753, .T. ) ;
#45510=ORIENTED_EDGE ( 'NONE', *, *, #26639, .F. ) ;
#45534=ORIENTED_EDGE ( 'NONE', *, *, #13121, .T. ) ;
#45546=LINE ( 'NONE', #5792, #14531 ) ;
#45578=CARTESIAN_POINT ( 'NONE',  ( 0.000000000000000000, 0.1473293504822046074, -0.9532488779249699284 ) ) ;
#45587=CARTESIAN_POINT ( 'NONE',  ( -0.3161444924769509779, 1.914733266569311532, -0.6843357808987579061 ) ) ;
#45590=CARTESIAN_POINT ( 'NONE',  ( -0.01585547164981869483, -0.5708661417322835607, 1.025733466389939119 ) ) ;
#45679=CARTESIAN_POINT ( 'NONE',  ( 0.1574803149606299746, 0.4265678656643324129, 0.4783464566929144235 ) ) ;
#45696=EDGE_CURVE ( 'NONE', #22261, #41308, #22904, .T. ) ;
#45698=CARTESIAN_POINT ( 'NONE',  ( -0.3161444924769509779, 2.177585298233989164, -4.122948637049707266 ) ) ;
#45706=DIRECTION ( 'NONE',  ( 0.000000000000000000, -0.7880107536067216811, 0.6156614753256587358 ) ) ;
#45750=VERTEX_POINT ( 'NONE', #34894 ) ;
#45825=CARTESIAN_POINT ( 'NONE',  ( 0.1574803149606299746, -0.5708661417322835607, 1.057384721142220263 ) ) ;
#45939=VERTEX_POINT ( 'NONE', #18068 ) ;
#45975=CIRCLE ( 'NONE', #1601, 0.2952755905511806334 ) ;
#46006=CIRCLE ( 'NONE', #33013, 0.2362204724409448231 ) ;
#46088=DIRECTION ( 'NONE',  ( 0.000000000000000000, 0.000000000000000000, 1.000000000000000000 ) ) ;
#46094=ORIENTED_EDGE ( 'NONE', *, *, #44329, .T. ) ;
#46104=CARTESIAN_POINT ( 'NONE',  ( -0.01585547164981869483, -0.5708661417322833387, 1.025733466389939119 ) ) ;
#46162=DIRECTION ( 'NONE',  ( 0.000000000000000000, 0.000000000000000000, -1.000000000000000000 ) ) ;
#46189=CARTESIAN_POINT ( 'NONE',  ( -0.1296641775163207277, 0.1169123912647608288, -2.121729632260068055 ) ) ;
#46229=DIRECTION ( 'NONE',  ( -1.000000000000000000, 0.000000000000000000, 0.000000000000000000 ) ) ;
#46267=VERTEX_POINT ( 'NONE', #539 ) ;
#46281=ORIENTED_EDGE ( 'NONE', *, *, #11885, .T. ) ;
#46304=AXIS2_PLACEMENT_3D ( 'NONE', #13421, #6200, #2145 ) ;
#46361=ADVANCED_FACE ( 'NONE', ( #24494 ), #13477, .F. ) ;
#46427=ORIENTED_EDGE ( 'NONE', *, *, #2320, .F. ) ;
#46478=CARTESIAN_POINT ( 'NONE',  ( -0.2834390116245509850, 0.3740157480314960647, 1.380828817464277991 ) ) ;
#46657=DIRECTION ( 'NONE',  ( -1.000000000000000000, 0.000000000000000000, 0.000000000000000000 ) ) ;
#46661=LINE ( 'NONE', #17438, #27754 ) ;
#46664=DIRECTION ( 'NONE',  ( 1.000000000000000000, -0.000000000000000000, -0.000000000000000000 ) ) ;
#46699=CARTESIAN_POINT ( 'NONE',  ( 0.1574803149606299746, 0.1473293504822046074, -0.9532488779249699284 ) ) ;
#46708=CARTESIAN_POINT ( 'NONE',  ( 0.06801279071809869514, -0.5708661417322835607, 1.224299699984025658 ) ) ;
#46711=CARTESIAN_POINT ( 'NONE',  ( 0.03901279071809810040, -0.09842519685039370636, 1.713085361781127913 ) ) ;
#46715=ORIENTED_EDGE ( 'NONE', *, *, #26648, .F. ) ;
#46747=ADVANCED_FACE ( 'NONE', ( #34016 ), #12439, .T. ) ;
#46758=DIRECTION ( 'NONE',  ( 0.000000000000000000, 9.251858538542967883E-16, 1.000000000000000000 ) ) ;
#46787=VERTEX_POINT ( 'NONE', #27303 ) ;
#46818=VECTOR ( 'NONE', #47391, 39.37007874015748143 ) ;
#46896=DIRECTION ( 'NONE',  ( 0.000000000000000000, 0.000000000000000000, -1.000000000000000000 ) ) ;
#47015=ORIENTED_EDGE ( 'NONE', *, *, #27301, .F. ) ;
#47026=EDGE_CURVE ( 'NONE', #39516, #11282, #8046, .T. ) ;
#47046=ORIENTED_EDGE ( 'NONE', *, *, #9491, .T. ) ;
#47057=EDGE_CURVE ( 'NONE', #23980, #13081, #36139, .T. ) ;
#47087=ORIENTED_EDGE ( 'NONE', *, *, #40660, .F. ) ;
#47118=EDGE_CURVE ( 'NONE', #7162, #33937, #18993, .T. ) ;
#47149=FACE_OUTER_BOUND ( 'NONE', #26061, .T. ) ;
#47151=LINE ( 'NONE', #13604, #46818 ) ;
#47198=EDGE_LOOP ( 'NONE', ( #37042, #31157, #45450, #32063 ) ) ;
#47199=DIRECTION ( 'NONE',  ( 0.000000000000000000, 0.000000000000000000, 1.000000000000000000 ) ) ;
#47296=CIRCLE ( 'NONE', #32778, 0.2362204724409448231 ) ;
#47327=EDGE_CURVE ( 'NONE', #14162, #44831, #5806, .T. ) ;
#47346=ORIENTED_EDGE ( 'NONE', *, *, #21354, .F. ) ;
#47350=EDGE_LOOP ( 'NONE', ( #25715, #11830, #21880, #40153 ) ) ;
#47358=EDGE_CURVE ( 'NONE', #45939, #31965, #6734, .T. ) ;
#47364=ORIENTED_EDGE ( 'NONE', *, *, #3268, .T. ) ;
#47391=DIRECTION ( 'NONE',  ( 5.934354299241488461E-32, 1.000000000000000000, 8.673617379884034486E-16 ) ) ;
#47403=VERTEX_POINT ( 'NONE', #9647 ) ;
ENDSEC;
END-ISO-10303-21;
